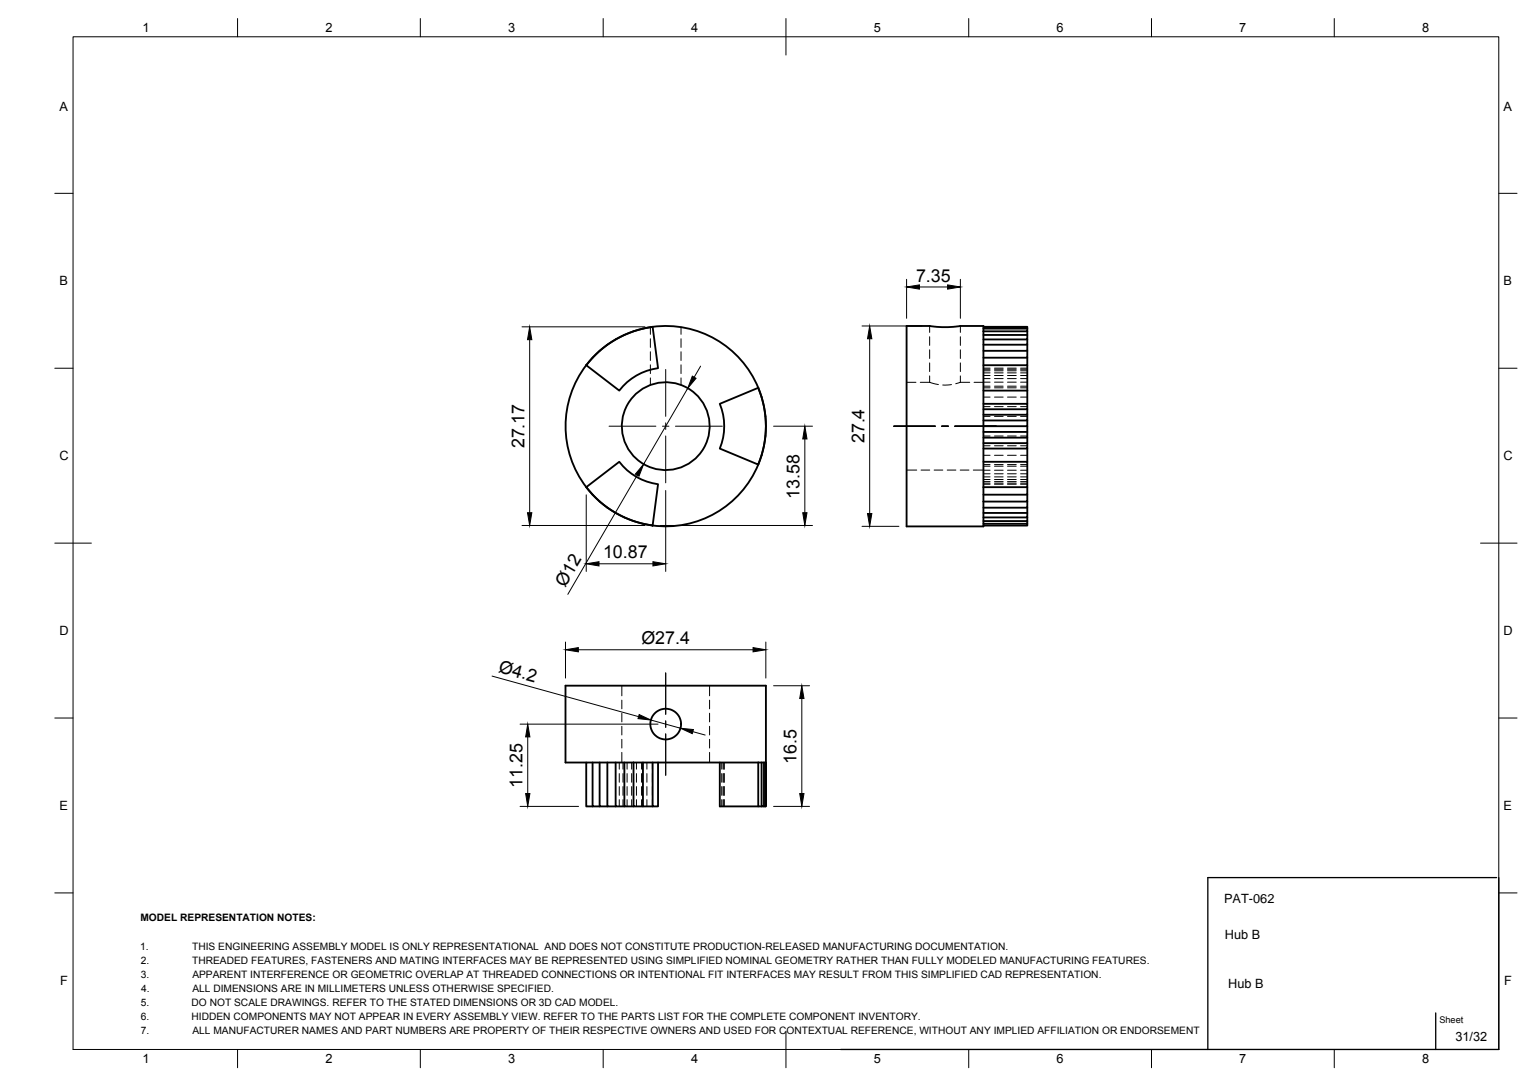
ISO-10303-21;
HEADER;
/* Generated by software containing ST-Developer
 * from STEP Tools, Inc. (www.steptools.com) 
 */

FILE_DESCRIPTION(
/* description */ ('Jaw-coupled motor to shaft test stand'),
/* implementation_level */ '2;1');

FILE_NAME(
/* name */ 'Hub B.step',
/* time_stamp */ '2026-10-27T10:46:06-07:00',
/* author */ (''),
/* organization */ (''),
/* preprocessor_version */ 'ST-DEVELOPER v20.2',
/* originating_system */ 'Autodesk Translation Framework v15.17.0.0',
/* authorisation */ '');

FILE_SCHEMA (('AUTOMOTIVE_DESIGN { 1 0 10303 214 3 1 1 }'));
ENDSEC;

DATA;
#10=MECHANICAL_DESIGN_GEOMETRIC_PRESENTATION_REPRESENTATION('',(#368),#19361);
#270=B_SPLINE_CURVE_WITH_KNOTS('',3,(#17784,#17785,#17786,#17787,#17788,
#17789,#17790,#17791,#17792,#17793,#17794,#17795,#17796,#17797,#17798,#17799,
#17800,#17801),.UNSPECIFIED.,.F.,.F.,(4,2,2,2,2,2,2,2,4),(0.,0.0798638474423531,
0.159727694884706,0.239545993340072,0.319364291795438,0.399182590250804,
0.47900088870617,0.558864736148523,0.638728583590876),.UNSPECIFIED.);
#271=B_SPLINE_CURVE_WITH_KNOTS('',3,(#17802,#17803,#17804,#17805,#17806,
#17807,#17808,#17809,#17810,#17811,#17812,#17813,#17814,#17815,#17816,#17817,
#17818,#17819),.UNSPECIFIED.,.F.,.F.,(4,2,2,2,2,2,2,2,4),(0.638728583590876,
0.718592431033229,0.798456278475583,0.878274576930949,0.958092875386314,
1.03791117384168,1.11772947229705,1.1975933197394,1.27745716718175),
 .UNSPECIFIED.);
#272=B_SPLINE_CURVE_WITH_KNOTS('',3,(#17823,#17824,#17825,#17826,#17827,
#17828,#17829,#17830,#17831,#17832,#17833,#17834,#17835,#17836,#17837,#17838,
#17839,#17840),.UNSPECIFIED.,.F.,.F.,(4,2,2,2,2,2,2,2,4),(0.,0.079239302416133,
0.158478604832266,0.237716399152057,0.316954193471848,0.39619198779164,
0.475429782111431,0.554669084527564,0.633908386943697),.UNSPECIFIED.);
#273=B_SPLINE_CURVE_WITH_KNOTS('',3,(#17841,#17842,#17843,#17844,#17845,
#17846,#17847,#17848,#17849,#17850,#17851,#17852,#17853,#17854,#17855,#17856,
#17857,#17858),.UNSPECIFIED.,.F.,.F.,(4,2,2,2,2,2,2,2,4),(0.633908386943697,
0.71314768935983,0.792386991775963,0.871624786095754,0.950862580415545,
1.03010037473534,1.10933816905513,1.18857747147126,1.26781677388739),
 .UNSPECIFIED.);
#303=SHAPE_REPRESENTATION_RELATIONSHIP('SRR','None',#19520,#335);
#335=ADVANCED_BREP_SHAPE_REPRESENTATION('',(#399),#19356);
#368=STYLED_ITEM('',(#19739),#399);
#399=MANIFOLD_SOLID_BREP('Body1',#11014);
#510=FACE_BOUND('',#2102,.T.);
#511=FACE_BOUND('',#2129,.T.);
#512=FACE_BOUND('',#2187,.T.);
#513=FACE_BOUND('',#2189,.T.);
#777=PLANE('',#11987);
#778=PLANE('',#11988);
#779=PLANE('',#11989);
#780=PLANE('',#11990);
#781=PLANE('',#11991);
#782=PLANE('',#11992);
#783=PLANE('',#11993);
#784=PLANE('',#11994);
#785=PLANE('',#11995);
#786=PLANE('',#11996);
#787=PLANE('',#11997);
#788=PLANE('',#11998);
#789=PLANE('',#11999);
#790=PLANE('',#12000);
#791=PLANE('',#12001);
#792=PLANE('',#12002);
#793=PLANE('',#12003);
#794=PLANE('',#12004);
#795=PLANE('',#12005);
#796=PLANE('',#12006);
#797=PLANE('',#12008);
#798=PLANE('',#12010);
#799=PLANE('',#12012);
#800=PLANE('',#12014);
#801=PLANE('',#12016);
#802=PLANE('',#12018);
#803=PLANE('',#12023);
#804=PLANE('',#12025);
#805=PLANE('',#12027);
#806=PLANE('',#12028);
#807=PLANE('',#12029);
#808=PLANE('',#12030);
#809=PLANE('',#12031);
#810=PLANE('',#12032);
#811=PLANE('',#12033);
#812=PLANE('',#12034);
#813=PLANE('',#12035);
#814=PLANE('',#12036);
#815=PLANE('',#12037);
#816=PLANE('',#12038);
#817=PLANE('',#12039);
#818=PLANE('',#12040);
#819=PLANE('',#12041);
#820=PLANE('',#12042);
#821=PLANE('',#12043);
#822=PLANE('',#12044);
#823=PLANE('',#12045);
#824=PLANE('',#12046);
#825=PLANE('',#12048);
#826=PLANE('',#12050);
#827=PLANE('',#12052);
#828=PLANE('',#12054);
#829=PLANE('',#12056);
#830=PLANE('',#12058);
#831=PLANE('',#12060);
#832=PLANE('',#12062);
#833=PLANE('',#12063);
#834=PLANE('',#12064);
#835=PLANE('',#12065);
#836=PLANE('',#12066);
#837=PLANE('',#12067);
#838=PLANE('',#12068);
#839=PLANE('',#12069);
#840=PLANE('',#12070);
#841=PLANE('',#12071);
#842=PLANE('',#12072);
#843=PLANE('',#12073);
#844=PLANE('',#12074);
#845=PLANE('',#12075);
#846=PLANE('',#12076);
#847=PLANE('',#12077);
#848=PLANE('',#12078);
#849=PLANE('',#12079);
#850=PLANE('',#12080);
#851=PLANE('',#12081);
#852=PLANE('',#12083);
#853=PLANE('',#12085);
#854=PLANE('',#12087);
#855=PLANE('',#12089);
#856=PLANE('',#12091);
#857=PLANE('',#12093);
#858=PLANE('',#12095);
#859=PLANE('',#12099);
#1373=FACE_OUTER_BOUND('',#2100,.T.);
#1374=FACE_OUTER_BOUND('',#2101,.T.);
#1375=FACE_OUTER_BOUND('',#2103,.T.);
#1376=FACE_OUTER_BOUND('',#2104,.T.);
#1377=FACE_OUTER_BOUND('',#2105,.T.);
#1378=FACE_OUTER_BOUND('',#2106,.T.);
#1379=FACE_OUTER_BOUND('',#2107,.T.);
#1380=FACE_OUTER_BOUND('',#2108,.T.);
#1381=FACE_OUTER_BOUND('',#2109,.T.);
#1382=FACE_OUTER_BOUND('',#2110,.T.);
#1383=FACE_OUTER_BOUND('',#2111,.T.);
#1384=FACE_OUTER_BOUND('',#2112,.T.);
#1385=FACE_OUTER_BOUND('',#2113,.T.);
#1386=FACE_OUTER_BOUND('',#2114,.T.);
#1387=FACE_OUTER_BOUND('',#2115,.T.);
#1388=FACE_OUTER_BOUND('',#2116,.T.);
#1389=FACE_OUTER_BOUND('',#2117,.T.);
#1390=FACE_OUTER_BOUND('',#2118,.T.);
#1391=FACE_OUTER_BOUND('',#2119,.T.);
#1392=FACE_OUTER_BOUND('',#2120,.T.);
#1393=FACE_OUTER_BOUND('',#2121,.T.);
#1394=FACE_OUTER_BOUND('',#2122,.T.);
#1395=FACE_OUTER_BOUND('',#2123,.T.);
#1396=FACE_OUTER_BOUND('',#2124,.T.);
#1397=FACE_OUTER_BOUND('',#2125,.T.);
#1398=FACE_OUTER_BOUND('',#2126,.T.);
#1399=FACE_OUTER_BOUND('',#2127,.T.);
#1400=FACE_OUTER_BOUND('',#2128,.T.);
#1401=FACE_OUTER_BOUND('',#2130,.T.);
#1402=FACE_OUTER_BOUND('',#2131,.T.);
#1403=FACE_OUTER_BOUND('',#2132,.T.);
#1404=FACE_OUTER_BOUND('',#2133,.T.);
#1405=FACE_OUTER_BOUND('',#2134,.T.);
#1406=FACE_OUTER_BOUND('',#2135,.T.);
#1407=FACE_OUTER_BOUND('',#2136,.T.);
#1408=FACE_OUTER_BOUND('',#2137,.T.);
#1409=FACE_OUTER_BOUND('',#2138,.T.);
#1410=FACE_OUTER_BOUND('',#2139,.T.);
#1411=FACE_OUTER_BOUND('',#2140,.T.);
#1412=FACE_OUTER_BOUND('',#2141,.T.);
#1413=FACE_OUTER_BOUND('',#2142,.T.);
#1414=FACE_OUTER_BOUND('',#2143,.T.);
#1415=FACE_OUTER_BOUND('',#2144,.T.);
#1416=FACE_OUTER_BOUND('',#2145,.T.);
#1417=FACE_OUTER_BOUND('',#2146,.T.);
#1418=FACE_OUTER_BOUND('',#2147,.T.);
#1419=FACE_OUTER_BOUND('',#2148,.T.);
#1420=FACE_OUTER_BOUND('',#2149,.T.);
#1421=FACE_OUTER_BOUND('',#2150,.T.);
#1422=FACE_OUTER_BOUND('',#2151,.T.);
#1423=FACE_OUTER_BOUND('',#2152,.T.);
#1424=FACE_OUTER_BOUND('',#2153,.T.);
#1425=FACE_OUTER_BOUND('',#2154,.T.);
#1426=FACE_OUTER_BOUND('',#2155,.T.);
#1427=FACE_OUTER_BOUND('',#2156,.T.);
#1428=FACE_OUTER_BOUND('',#2157,.T.);
#1429=FACE_OUTER_BOUND('',#2158,.T.);
#1430=FACE_OUTER_BOUND('',#2159,.T.);
#1431=FACE_OUTER_BOUND('',#2160,.T.);
#1432=FACE_OUTER_BOUND('',#2161,.T.);
#1433=FACE_OUTER_BOUND('',#2162,.T.);
#1434=FACE_OUTER_BOUND('',#2163,.T.);
#1435=FACE_OUTER_BOUND('',#2164,.T.);
#1436=FACE_OUTER_BOUND('',#2165,.T.);
#1437=FACE_OUTER_BOUND('',#2166,.T.);
#1438=FACE_OUTER_BOUND('',#2167,.T.);
#1439=FACE_OUTER_BOUND('',#2168,.T.);
#1440=FACE_OUTER_BOUND('',#2169,.T.);
#1441=FACE_OUTER_BOUND('',#2170,.T.);
#1442=FACE_OUTER_BOUND('',#2171,.T.);
#1443=FACE_OUTER_BOUND('',#2172,.T.);
#1444=FACE_OUTER_BOUND('',#2173,.T.);
#1445=FACE_OUTER_BOUND('',#2174,.T.);
#1446=FACE_OUTER_BOUND('',#2175,.T.);
#1447=FACE_OUTER_BOUND('',#2176,.T.);
#1448=FACE_OUTER_BOUND('',#2177,.T.);
#1449=FACE_OUTER_BOUND('',#2178,.T.);
#1450=FACE_OUTER_BOUND('',#2179,.T.);
#1451=FACE_OUTER_BOUND('',#2180,.T.);
#1452=FACE_OUTER_BOUND('',#2181,.T.);
#1453=FACE_OUTER_BOUND('',#2182,.T.);
#1454=FACE_OUTER_BOUND('',#2183,.T.);
#1455=FACE_OUTER_BOUND('',#2184,.T.);
#1456=FACE_OUTER_BOUND('',#2185,.T.);
#1457=FACE_OUTER_BOUND('',#2186,.T.);
#1458=FACE_OUTER_BOUND('',#2188,.T.);
#2100=EDGE_LOOP('',(#8872,#8873,#8874,#8875,#8876,#8877));
#2101=EDGE_LOOP('',(#8878,#8879,#8880,#8881));
#2102=EDGE_LOOP('',(#8882,#8883));
#2103=EDGE_LOOP('',(#8884,#8885,#8886,#8887));
#2104=EDGE_LOOP('',(#8888,#8889,#8890,#8891));
#2105=EDGE_LOOP('',(#8892,#8893,#8894,#8895));
#2106=EDGE_LOOP('',(#8896,#8897,#8898,#8899));
#2107=EDGE_LOOP('',(#8900,#8901,#8902,#8903));
#2108=EDGE_LOOP('',(#8904,#8905,#8906,#8907));
#2109=EDGE_LOOP('',(#8908,#8909,#8910,#8911));
#2110=EDGE_LOOP('',(#8912,#8913,#8914,#8915));
#2111=EDGE_LOOP('',(#8916,#8917,#8918,#8919));
#2112=EDGE_LOOP('',(#8920,#8921,#8922,#8923));
#2113=EDGE_LOOP('',(#8924,#8925,#8926,#8927));
#2114=EDGE_LOOP('',(#8928,#8929,#8930,#8931));
#2115=EDGE_LOOP('',(#8932,#8933,#8934,#8935));
#2116=EDGE_LOOP('',(#8936,#8937,#8938,#8939));
#2117=EDGE_LOOP('',(#8940,#8941,#8942,#8943));
#2118=EDGE_LOOP('',(#8944,#8945,#8946,#8947));
#2119=EDGE_LOOP('',(#8948,#8949,#8950,#8951));
#2120=EDGE_LOOP('',(#8952,#8953,#8954,#8955));
#2121=EDGE_LOOP('',(#8956,#8957,#8958,#8959,#8960,#8961,#8962,#8963,#8964,
#8965,#8966,#8967,#8968,#8969,#8970,#8971,#8972,#8973));
#2122=EDGE_LOOP('',(#8974,#8975));
#2123=EDGE_LOOP('',(#8976,#8977));
#2124=EDGE_LOOP('',(#8978,#8979));
#2125=EDGE_LOOP('',(#8980,#8981));
#2126=EDGE_LOOP('',(#8982,#8983));
#2127=EDGE_LOOP('',(#8984,#8985));
#2128=EDGE_LOOP('',(#8986,#8987,#8988,#8989,#8990,#8991,#8992,#8993,#8994,
#8995,#8996,#8997,#8998,#8999,#9000,#9001,#9002,#9003,#9004,#9005,#9006,
#9007,#9008,#9009,#9010,#9011,#9012,#9013,#9014,#9015,#9016,#9017,#9018,
#9019));
#2129=EDGE_LOOP('',(#9020));
#2130=EDGE_LOOP('',(#9021,#9022));
#2131=EDGE_LOOP('',(#9023,#9024));
#2132=EDGE_LOOP('',(#9025,#9026,#9027,#9028));
#2133=EDGE_LOOP('',(#9029,#9030,#9031,#9032));
#2134=EDGE_LOOP('',(#9033,#9034,#9035,#9036));
#2135=EDGE_LOOP('',(#9037,#9038,#9039,#9040));
#2136=EDGE_LOOP('',(#9041,#9042,#9043,#9044));
#2137=EDGE_LOOP('',(#9045,#9046,#9047,#9048));
#2138=EDGE_LOOP('',(#9049,#9050,#9051,#9052));
#2139=EDGE_LOOP('',(#9053,#9054,#9055,#9056));
#2140=EDGE_LOOP('',(#9057,#9058,#9059,#9060));
#2141=EDGE_LOOP('',(#9061,#9062,#9063,#9064));
#2142=EDGE_LOOP('',(#9065,#9066,#9067,#9068));
#2143=EDGE_LOOP('',(#9069,#9070,#9071,#9072));
#2144=EDGE_LOOP('',(#9073,#9074,#9075,#9076));
#2145=EDGE_LOOP('',(#9077,#9078,#9079,#9080));
#2146=EDGE_LOOP('',(#9081,#9082,#9083,#9084));
#2147=EDGE_LOOP('',(#9085,#9086,#9087,#9088));
#2148=EDGE_LOOP('',(#9089,#9090,#9091,#9092));
#2149=EDGE_LOOP('',(#9093,#9094,#9095,#9096));
#2150=EDGE_LOOP('',(#9097,#9098,#9099,#9100,#9101,#9102,#9103,#9104,#9105,
#9106,#9107,#9108,#9109,#9110,#9111,#9112,#9113,#9114));
#2151=EDGE_LOOP('',(#9115,#9116));
#2152=EDGE_LOOP('',(#9117,#9118));
#2153=EDGE_LOOP('',(#9119,#9120));
#2154=EDGE_LOOP('',(#9121,#9122));
#2155=EDGE_LOOP('',(#9123,#9124));
#2156=EDGE_LOOP('',(#9125,#9126));
#2157=EDGE_LOOP('',(#9127,#9128));
#2158=EDGE_LOOP('',(#9129,#9130));
#2159=EDGE_LOOP('',(#9131,#9132,#9133,#9134));
#2160=EDGE_LOOP('',(#9135,#9136,#9137,#9138));
#2161=EDGE_LOOP('',(#9139,#9140,#9141,#9142));
#2162=EDGE_LOOP('',(#9143,#9144,#9145,#9146));
#2163=EDGE_LOOP('',(#9147,#9148,#9149,#9150));
#2164=EDGE_LOOP('',(#9151,#9152,#9153,#9154));
#2165=EDGE_LOOP('',(#9155,#9156,#9157,#9158));
#2166=EDGE_LOOP('',(#9159,#9160,#9161,#9162));
#2167=EDGE_LOOP('',(#9163,#9164,#9165,#9166));
#2168=EDGE_LOOP('',(#9167,#9168,#9169,#9170));
#2169=EDGE_LOOP('',(#9171,#9172,#9173,#9174));
#2170=EDGE_LOOP('',(#9175,#9176,#9177,#9178));
#2171=EDGE_LOOP('',(#9179,#9180,#9181,#9182));
#2172=EDGE_LOOP('',(#9183,#9184,#9185,#9186));
#2173=EDGE_LOOP('',(#9187,#9188,#9189,#9190));
#2174=EDGE_LOOP('',(#9191,#9192,#9193,#9194));
#2175=EDGE_LOOP('',(#9195,#9196,#9197,#9198));
#2176=EDGE_LOOP('',(#9199,#9200,#9201,#9202));
#2177=EDGE_LOOP('',(#9203,#9204,#9205,#9206,#9207,#9208,#9209,#9210,#9211,
#9212,#9213,#9214,#9215,#9216,#9217,#9218,#9219,#9220));
#2178=EDGE_LOOP('',(#9221,#9222));
#2179=EDGE_LOOP('',(#9223,#9224));
#2180=EDGE_LOOP('',(#9225,#9226));
#2181=EDGE_LOOP('',(#9227,#9228));
#2182=EDGE_LOOP('',(#9229,#9230));
#2183=EDGE_LOOP('',(#9231,#9232));
#2184=EDGE_LOOP('',(#9233,#9234));
#2185=EDGE_LOOP('',(#9235,#9236));
#2186=EDGE_LOOP('',(#9237,#9238,#9239,#9240,#9241,#9242,#9243,#9244,#9245,
#9246,#9247,#9248,#9249,#9250,#9251,#9252,#9253,#9254,#9255,#9256,#9257,
#9258,#9259,#9260,#9261,#9262,#9263,#9264,#9265,#9266,#9267));
#2187=EDGE_LOOP('',(#9268,#9269));
#2188=EDGE_LOOP('',(#9270));
#2189=EDGE_LOOP('',(#9271));
#2896=LINE('',#17821,#4049);
#2897=LINE('',#17863,#4050);
#2898=LINE('',#17868,#4051);
#2899=LINE('',#17870,#4052);
#2900=LINE('',#17872,#4053);
#2901=LINE('',#17873,#4054);
#2902=LINE('',#17876,#4055);
#2903=LINE('',#17878,#4056);
#2904=LINE('',#17879,#4057);
#2905=LINE('',#17882,#4058);
#2906=LINE('',#17884,#4059);
#2907=LINE('',#17885,#4060);
#2908=LINE('',#17888,#4061);
#2909=LINE('',#17890,#4062);
#2910=LINE('',#17891,#4063);
#2911=LINE('',#17894,#4064);
#2912=LINE('',#17896,#4065);
#2913=LINE('',#17897,#4066);
#2914=LINE('',#17900,#4067);
#2915=LINE('',#17902,#4068);
#2916=LINE('',#17903,#4069);
#2917=LINE('',#17906,#4070);
#2918=LINE('',#17908,#4071);
#2919=LINE('',#17909,#4072);
#2920=LINE('',#17912,#4073);
#2921=LINE('',#17914,#4074);
#2922=LINE('',#17915,#4075);
#2923=LINE('',#17918,#4076);
#2924=LINE('',#17920,#4077);
#2925=LINE('',#17921,#4078);
#2926=LINE('',#17924,#4079);
#2927=LINE('',#17926,#4080);
#2928=LINE('',#17927,#4081);
#2929=LINE('',#17930,#4082);
#2930=LINE('',#17932,#4083);
#2931=LINE('',#17933,#4084);
#2932=LINE('',#17936,#4085);
#2933=LINE('',#17938,#4086);
#2934=LINE('',#17939,#4087);
#2935=LINE('',#17942,#4088);
#2936=LINE('',#17944,#4089);
#2937=LINE('',#17945,#4090);
#2938=LINE('',#17948,#4091);
#2939=LINE('',#17950,#4092);
#2940=LINE('',#17951,#4093);
#2941=LINE('',#17954,#4094);
#2942=LINE('',#17956,#4095);
#2943=LINE('',#17957,#4096);
#2944=LINE('',#17960,#4097);
#2945=LINE('',#17962,#4098);
#2946=LINE('',#17963,#4099);
#2947=LINE('',#17966,#4100);
#2948=LINE('',#17968,#4101);
#2949=LINE('',#17969,#4102);
#2950=LINE('',#17971,#4103);
#2951=LINE('',#17972,#4104);
#2952=LINE('',#17992,#4105);
#2953=LINE('',#17994,#4106);
#2954=LINE('',#17996,#4107);
#2955=LINE('',#17998,#4108);
#2956=LINE('',#18000,#4109);
#2957=LINE('',#18002,#4110);
#2958=LINE('',#18004,#4111);
#2959=LINE('',#18006,#4112);
#2960=LINE('',#18008,#4113);
#2961=LINE('',#18010,#4114);
#2962=LINE('',#18014,#4115);
#2963=LINE('',#18016,#4116);
#2964=LINE('',#18018,#4117);
#2965=LINE('',#18020,#4118);
#2966=LINE('',#18022,#4119);
#2967=LINE('',#18024,#4120);
#2968=LINE('',#18026,#4121);
#2969=LINE('',#18028,#4122);
#2970=LINE('',#18030,#4123);
#2971=LINE('',#18032,#4124);
#2972=LINE('',#18041,#4125);
#2973=LINE('',#18042,#4126);
#2974=LINE('',#18043,#4127);
#2975=LINE('',#18046,#4128);
#2976=LINE('',#18047,#4129);
#2977=LINE('',#18050,#4130);
#2978=LINE('',#18051,#4131);
#2979=LINE('',#18054,#4132);
#2980=LINE('',#18055,#4133);
#2981=LINE('',#18058,#4134);
#2982=LINE('',#18059,#4135);
#2983=LINE('',#18062,#4136);
#2984=LINE('',#18063,#4137);
#2985=LINE('',#18066,#4138);
#2986=LINE('',#18067,#4139);
#2987=LINE('',#18070,#4140);
#2988=LINE('',#18071,#4141);
#2989=LINE('',#18074,#4142);
#2990=LINE('',#18075,#4143);
#2991=LINE('',#18078,#4144);
#2992=LINE('',#18080,#4145);
#2993=LINE('',#18081,#4146);
#2994=LINE('',#18084,#4147);
#2995=LINE('',#18086,#4148);
#2996=LINE('',#18087,#4149);
#2997=LINE('',#18090,#4150);
#2998=LINE('',#18092,#4151);
#2999=LINE('',#18093,#4152);
#3000=LINE('',#18096,#4153);
#3001=LINE('',#18098,#4154);
#3002=LINE('',#18099,#4155);
#3003=LINE('',#18102,#4156);
#3004=LINE('',#18104,#4157);
#3005=LINE('',#18105,#4158);
#3006=LINE('',#18108,#4159);
#3007=LINE('',#18110,#4160);
#3008=LINE('',#18111,#4161);
#3009=LINE('',#18114,#4162);
#3010=LINE('',#18116,#4163);
#3011=LINE('',#18117,#4164);
#3012=LINE('',#18120,#4165);
#3013=LINE('',#18121,#4166);
#3014=LINE('',#18122,#4167);
#3015=LINE('',#18124,#4168);
#3016=LINE('',#18145,#4169);
#3017=LINE('',#18146,#4170);
#3018=LINE('',#18147,#4171);
#3019=LINE('',#18150,#4172);
#3020=LINE('',#18151,#4173);
#3021=LINE('',#18154,#4174);
#3022=LINE('',#18155,#4175);
#3023=LINE('',#18158,#4176);
#3024=LINE('',#18159,#4177);
#3025=LINE('',#18162,#4178);
#3026=LINE('',#18163,#4179);
#3027=LINE('',#18166,#4180);
#3028=LINE('',#18167,#4181);
#3029=LINE('',#18170,#4182);
#3030=LINE('',#18171,#4183);
#3031=LINE('',#18174,#4184);
#3032=LINE('',#18175,#4185);
#3033=LINE('',#18178,#4186);
#3034=LINE('',#18179,#4187);
#3035=LINE('',#18182,#4188);
#3036=LINE('',#18184,#4189);
#3037=LINE('',#18185,#4190);
#3038=LINE('',#18188,#4191);
#3039=LINE('',#18190,#4192);
#3040=LINE('',#18191,#4193);
#3041=LINE('',#18194,#4194);
#3042=LINE('',#18196,#4195);
#3043=LINE('',#18197,#4196);
#3044=LINE('',#18200,#4197);
#3045=LINE('',#18202,#4198);
#3046=LINE('',#18203,#4199);
#3047=LINE('',#18206,#4200);
#3048=LINE('',#18208,#4201);
#3049=LINE('',#18209,#4202);
#3050=LINE('',#18212,#4203);
#3051=LINE('',#18214,#4204);
#3052=LINE('',#18215,#4205);
#3053=LINE('',#18218,#4206);
#3054=LINE('',#18220,#4207);
#3055=LINE('',#18221,#4208);
#3056=LINE('',#18224,#4209);
#3057=LINE('',#18225,#4210);
#3058=LINE('',#18226,#4211);
#3059=LINE('',#18228,#4212);
#3060=LINE('',#18249,#4213);
#4049=VECTOR('',#14083,0.21);
#4050=VECTOR('',#14088,0.6);
#4051=VECTOR('',#14093,1.);
#4052=VECTOR('',#14094,1.);
#4053=VECTOR('',#14095,1.);
#4054=VECTOR('',#14096,1.);
#4055=VECTOR('',#14099,1.);
#4056=VECTOR('',#14100,1.);
#4057=VECTOR('',#14101,1.);
#4058=VECTOR('',#14104,1.);
#4059=VECTOR('',#14105,1.);
#4060=VECTOR('',#14106,1.);
#4061=VECTOR('',#14109,1.);
#4062=VECTOR('',#14110,1.);
#4063=VECTOR('',#14111,1.);
#4064=VECTOR('',#14114,1.);
#4065=VECTOR('',#14115,1.);
#4066=VECTOR('',#14116,1.);
#4067=VECTOR('',#14119,1.);
#4068=VECTOR('',#14120,1.);
#4069=VECTOR('',#14121,1.);
#4070=VECTOR('',#14124,1.);
#4071=VECTOR('',#14125,1.);
#4072=VECTOR('',#14126,1.);
#4073=VECTOR('',#14129,1.);
#4074=VECTOR('',#14130,1.);
#4075=VECTOR('',#14131,1.);
#4076=VECTOR('',#14134,1.);
#4077=VECTOR('',#14135,1.);
#4078=VECTOR('',#14136,1.);
#4079=VECTOR('',#14139,1.);
#4080=VECTOR('',#14140,1.);
#4081=VECTOR('',#14141,1.);
#4082=VECTOR('',#14144,1.);
#4083=VECTOR('',#14145,1.);
#4084=VECTOR('',#14146,1.);
#4085=VECTOR('',#14149,1.);
#4086=VECTOR('',#14150,1.);
#4087=VECTOR('',#14151,1.);
#4088=VECTOR('',#14154,1.);
#4089=VECTOR('',#14155,1.);
#4090=VECTOR('',#14156,1.);
#4091=VECTOR('',#14159,1.);
#4092=VECTOR('',#14160,1.);
#4093=VECTOR('',#14161,1.);
#4094=VECTOR('',#14164,1.);
#4095=VECTOR('',#14165,1.);
#4096=VECTOR('',#14166,1.);
#4097=VECTOR('',#14169,1.);
#4098=VECTOR('',#14170,1.);
#4099=VECTOR('',#14171,1.);
#4100=VECTOR('',#14174,1.);
#4101=VECTOR('',#14175,1.);
#4102=VECTOR('',#14176,1.);
#4103=VECTOR('',#14179,1.);
#4104=VECTOR('',#14180,1.);
#4105=VECTOR('',#14213,1.);
#4106=VECTOR('',#14214,1.);
#4107=VECTOR('',#14215,1.);
#4108=VECTOR('',#14216,1.);
#4109=VECTOR('',#14217,1.);
#4110=VECTOR('',#14218,1.);
#4111=VECTOR('',#14219,1.);
#4112=VECTOR('',#14220,1.);
#4113=VECTOR('',#14221,1.);
#4114=VECTOR('',#14222,1.);
#4115=VECTOR('',#14225,1.);
#4116=VECTOR('',#14226,1.);
#4117=VECTOR('',#14227,1.);
#4118=VECTOR('',#14228,1.);
#4119=VECTOR('',#14229,1.);
#4120=VECTOR('',#14230,1.);
#4121=VECTOR('',#14231,1.);
#4122=VECTOR('',#14232,1.);
#4123=VECTOR('',#14233,1.);
#4124=VECTOR('',#14234,1.);
#4125=VECTOR('',#14247,1.);
#4126=VECTOR('',#14248,1.);
#4127=VECTOR('',#14249,1.);
#4128=VECTOR('',#14252,1.);
#4129=VECTOR('',#14253,1.);
#4130=VECTOR('',#14256,1.);
#4131=VECTOR('',#14257,1.);
#4132=VECTOR('',#14260,1.);
#4133=VECTOR('',#14261,1.);
#4134=VECTOR('',#14264,1.);
#4135=VECTOR('',#14265,1.);
#4136=VECTOR('',#14268,1.);
#4137=VECTOR('',#14269,1.);
#4138=VECTOR('',#14272,1.);
#4139=VECTOR('',#14273,1.);
#4140=VECTOR('',#14276,1.);
#4141=VECTOR('',#14277,1.);
#4142=VECTOR('',#14280,1.);
#4143=VECTOR('',#14281,1.);
#4144=VECTOR('',#14284,1.);
#4145=VECTOR('',#14285,1.);
#4146=VECTOR('',#14286,1.);
#4147=VECTOR('',#14289,1.);
#4148=VECTOR('',#14290,1.);
#4149=VECTOR('',#14291,1.);
#4150=VECTOR('',#14294,1.);
#4151=VECTOR('',#14295,1.);
#4152=VECTOR('',#14296,1.);
#4153=VECTOR('',#14299,1.);
#4154=VECTOR('',#14300,1.);
#4155=VECTOR('',#14301,1.);
#4156=VECTOR('',#14304,1.);
#4157=VECTOR('',#14305,1.);
#4158=VECTOR('',#14306,1.);
#4159=VECTOR('',#14309,1.);
#4160=VECTOR('',#14310,1.);
#4161=VECTOR('',#14311,1.);
#4162=VECTOR('',#14314,1.);
#4163=VECTOR('',#14315,1.);
#4164=VECTOR('',#14316,1.);
#4165=VECTOR('',#14319,1.);
#4166=VECTOR('',#14320,1.);
#4167=VECTOR('',#14321,1.);
#4168=VECTOR('',#14324,1.);
#4169=VECTOR('',#14361,1.);
#4170=VECTOR('',#14362,1.);
#4171=VECTOR('',#14363,1.);
#4172=VECTOR('',#14366,1.);
#4173=VECTOR('',#14367,1.);
#4174=VECTOR('',#14370,1.);
#4175=VECTOR('',#14371,1.);
#4176=VECTOR('',#14374,1.);
#4177=VECTOR('',#14375,1.);
#4178=VECTOR('',#14378,1.);
#4179=VECTOR('',#14379,1.);
#4180=VECTOR('',#14382,1.);
#4181=VECTOR('',#14383,1.);
#4182=VECTOR('',#14386,1.);
#4183=VECTOR('',#14387,1.);
#4184=VECTOR('',#14390,1.);
#4185=VECTOR('',#14391,1.);
#4186=VECTOR('',#14394,1.);
#4187=VECTOR('',#14395,1.);
#4188=VECTOR('',#14398,1.);
#4189=VECTOR('',#14399,1.);
#4190=VECTOR('',#14400,1.);
#4191=VECTOR('',#14403,1.);
#4192=VECTOR('',#14404,1.);
#4193=VECTOR('',#14405,1.);
#4194=VECTOR('',#14408,1.);
#4195=VECTOR('',#14409,1.);
#4196=VECTOR('',#14410,1.);
#4197=VECTOR('',#14413,1.);
#4198=VECTOR('',#14414,1.);
#4199=VECTOR('',#14415,1.);
#4200=VECTOR('',#14418,1.);
#4201=VECTOR('',#14419,1.);
#4202=VECTOR('',#14420,1.);
#4203=VECTOR('',#14423,1.);
#4204=VECTOR('',#14424,1.);
#4205=VECTOR('',#14425,1.);
#4206=VECTOR('',#14428,1.);
#4207=VECTOR('',#14429,1.);
#4208=VECTOR('',#14430,1.);
#4209=VECTOR('',#14433,1.);
#4210=VECTOR('',#14434,1.);
#4211=VECTOR('',#14435,1.);
#4212=VECTOR('',#14438,1.);
#4213=VECTOR('',#14477,1.37);
#4880=CIRCLE('',#11985,0.6);
#4881=CIRCLE('',#11986,0.6);
#4882=CIRCLE('',#12007,1.37);
#4883=CIRCLE('',#12009,1.37);
#4884=CIRCLE('',#12011,1.37);
#4885=CIRCLE('',#12013,1.37);
#4886=CIRCLE('',#12015,1.37);
#4887=CIRCLE('',#12017,1.37);
#4888=CIRCLE('',#12019,1.37);
#4889=CIRCLE('',#12020,1.37);
#4890=CIRCLE('',#12021,1.37);
#4891=CIRCLE('',#12022,1.37);
#4892=CIRCLE('',#12024,1.37);
#4893=CIRCLE('',#12026,1.37);
#4894=CIRCLE('',#12047,1.37);
#4895=CIRCLE('',#12049,1.37);
#4896=CIRCLE('',#12051,1.37);
#4897=CIRCLE('',#12053,1.37);
#4898=CIRCLE('',#12055,1.37);
#4899=CIRCLE('',#12057,1.37);
#4900=CIRCLE('',#12059,1.37);
#4901=CIRCLE('',#12061,1.37);
#4902=CIRCLE('',#12082,1.37);
#4903=CIRCLE('',#12084,1.37);
#4904=CIRCLE('',#12086,1.37);
#4905=CIRCLE('',#12088,1.37);
#4906=CIRCLE('',#12090,1.37);
#4907=CIRCLE('',#12092,1.37);
#4908=CIRCLE('',#12094,1.37);
#4909=CIRCLE('',#12096,1.37);
#4910=CIRCLE('',#12098,1.37);
#5440=VERTEX_POINT('',#17782);
#5441=VERTEX_POINT('',#17783);
#5442=VERTEX_POINT('',#17820);
#5443=VERTEX_POINT('',#17822);
#5444=VERTEX_POINT('',#17860);
#5445=VERTEX_POINT('',#17862);
#5446=VERTEX_POINT('',#17866);
#5447=VERTEX_POINT('',#17867);
#5448=VERTEX_POINT('',#17869);
#5449=VERTEX_POINT('',#17871);
#5450=VERTEX_POINT('',#17875);
#5451=VERTEX_POINT('',#17877);
#5452=VERTEX_POINT('',#17881);
#5453=VERTEX_POINT('',#17883);
#5454=VERTEX_POINT('',#17887);
#5455=VERTEX_POINT('',#17889);
#5456=VERTEX_POINT('',#17893);
#5457=VERTEX_POINT('',#17895);
#5458=VERTEX_POINT('',#17899);
#5459=VERTEX_POINT('',#17901);
#5460=VERTEX_POINT('',#17905);
#5461=VERTEX_POINT('',#17907);
#5462=VERTEX_POINT('',#17911);
#5463=VERTEX_POINT('',#17913);
#5464=VERTEX_POINT('',#17917);
#5465=VERTEX_POINT('',#17919);
#5466=VERTEX_POINT('',#17923);
#5467=VERTEX_POINT('',#17925);
#5468=VERTEX_POINT('',#17929);
#5469=VERTEX_POINT('',#17931);
#5470=VERTEX_POINT('',#17935);
#5471=VERTEX_POINT('',#17937);
#5472=VERTEX_POINT('',#17941);
#5473=VERTEX_POINT('',#17943);
#5474=VERTEX_POINT('',#17947);
#5475=VERTEX_POINT('',#17949);
#5476=VERTEX_POINT('',#17953);
#5477=VERTEX_POINT('',#17955);
#5478=VERTEX_POINT('',#17959);
#5479=VERTEX_POINT('',#17961);
#5480=VERTEX_POINT('',#17965);
#5481=VERTEX_POINT('',#17967);
#5482=VERTEX_POINT('',#17987);
#5483=VERTEX_POINT('',#17989);
#5484=VERTEX_POINT('',#17991);
#5485=VERTEX_POINT('',#17993);
#5486=VERTEX_POINT('',#17995);
#5487=VERTEX_POINT('',#17997);
#5488=VERTEX_POINT('',#17999);
#5489=VERTEX_POINT('',#18001);
#5490=VERTEX_POINT('',#18003);
#5491=VERTEX_POINT('',#18005);
#5492=VERTEX_POINT('',#18007);
#5493=VERTEX_POINT('',#18009);
#5494=VERTEX_POINT('',#18011);
#5495=VERTEX_POINT('',#18013);
#5496=VERTEX_POINT('',#18015);
#5497=VERTEX_POINT('',#18017);
#5498=VERTEX_POINT('',#18019);
#5499=VERTEX_POINT('',#18021);
#5500=VERTEX_POINT('',#18023);
#5501=VERTEX_POINT('',#18025);
#5502=VERTEX_POINT('',#18027);
#5503=VERTEX_POINT('',#18029);
#5504=VERTEX_POINT('',#18031);
#5505=VERTEX_POINT('',#18039);
#5506=VERTEX_POINT('',#18040);
#5507=VERTEX_POINT('',#18045);
#5508=VERTEX_POINT('',#18049);
#5509=VERTEX_POINT('',#18053);
#5510=VERTEX_POINT('',#18057);
#5511=VERTEX_POINT('',#18061);
#5512=VERTEX_POINT('',#18065);
#5513=VERTEX_POINT('',#18069);
#5514=VERTEX_POINT('',#18073);
#5515=VERTEX_POINT('',#18077);
#5516=VERTEX_POINT('',#18079);
#5517=VERTEX_POINT('',#18083);
#5518=VERTEX_POINT('',#18085);
#5519=VERTEX_POINT('',#18089);
#5520=VERTEX_POINT('',#18091);
#5521=VERTEX_POINT('',#18095);
#5522=VERTEX_POINT('',#18097);
#5523=VERTEX_POINT('',#18101);
#5524=VERTEX_POINT('',#18103);
#5525=VERTEX_POINT('',#18107);
#5526=VERTEX_POINT('',#18109);
#5527=VERTEX_POINT('',#18113);
#5528=VERTEX_POINT('',#18115);
#5529=VERTEX_POINT('',#18119);
#5530=VERTEX_POINT('',#18143);
#5531=VERTEX_POINT('',#18144);
#5532=VERTEX_POINT('',#18149);
#5533=VERTEX_POINT('',#18153);
#5534=VERTEX_POINT('',#18157);
#5535=VERTEX_POINT('',#18161);
#5536=VERTEX_POINT('',#18165);
#5537=VERTEX_POINT('',#18169);
#5538=VERTEX_POINT('',#18173);
#5539=VERTEX_POINT('',#18177);
#5540=VERTEX_POINT('',#18181);
#5541=VERTEX_POINT('',#18183);
#5542=VERTEX_POINT('',#18187);
#5543=VERTEX_POINT('',#18189);
#5544=VERTEX_POINT('',#18193);
#5545=VERTEX_POINT('',#18195);
#5546=VERTEX_POINT('',#18199);
#5547=VERTEX_POINT('',#18201);
#5548=VERTEX_POINT('',#18205);
#5549=VERTEX_POINT('',#18207);
#5550=VERTEX_POINT('',#18211);
#5551=VERTEX_POINT('',#18213);
#5552=VERTEX_POINT('',#18217);
#5553=VERTEX_POINT('',#18219);
#5554=VERTEX_POINT('',#18223);
#5555=VERTEX_POINT('',#18247);
#6647=EDGE_CURVE('',#5440,#5441,#270,.T.);
#6648=EDGE_CURVE('',#5441,#5440,#271,.T.);
#6649=EDGE_CURVE('',#5441,#5442,#2896,.T.);
#6650=EDGE_CURVE('',#5443,#5442,#272,.T.);
#6651=EDGE_CURVE('',#5442,#5443,#273,.T.);
#6652=EDGE_CURVE('',#5444,#5444,#4880,.T.);
#6653=EDGE_CURVE('',#5444,#5445,#2897,.T.);
#6654=EDGE_CURVE('',#5445,#5445,#4881,.T.);
#6655=EDGE_CURVE('',#5446,#5447,#2898,.T.);
#6656=EDGE_CURVE('',#5447,#5448,#2899,.T.);
#6657=EDGE_CURVE('',#5449,#5448,#2900,.T.);
#6658=EDGE_CURVE('',#5446,#5449,#2901,.T.);
#6659=EDGE_CURVE('',#5450,#5446,#2902,.T.);
#6660=EDGE_CURVE('',#5451,#5449,#2903,.T.);
#6661=EDGE_CURVE('',#5450,#5451,#2904,.T.);
#6662=EDGE_CURVE('',#5452,#5450,#2905,.T.);
#6663=EDGE_CURVE('',#5453,#5451,#2906,.T.);
#6664=EDGE_CURVE('',#5452,#5453,#2907,.T.);
#6665=EDGE_CURVE('',#5454,#5452,#2908,.T.);
#6666=EDGE_CURVE('',#5455,#5453,#2909,.T.);
#6667=EDGE_CURVE('',#5454,#5455,#2910,.T.);
#6668=EDGE_CURVE('',#5456,#5454,#2911,.T.);
#6669=EDGE_CURVE('',#5457,#5455,#2912,.T.);
#6670=EDGE_CURVE('',#5456,#5457,#2913,.T.);
#6671=EDGE_CURVE('',#5458,#5456,#2914,.T.);
#6672=EDGE_CURVE('',#5459,#5457,#2915,.T.);
#6673=EDGE_CURVE('',#5458,#5459,#2916,.T.);
#6674=EDGE_CURVE('',#5460,#5458,#2917,.T.);
#6675=EDGE_CURVE('',#5461,#5459,#2918,.T.);
#6676=EDGE_CURVE('',#5460,#5461,#2919,.T.);
#6677=EDGE_CURVE('',#5462,#5460,#2920,.T.);
#6678=EDGE_CURVE('',#5463,#5461,#2921,.T.);
#6679=EDGE_CURVE('',#5462,#5463,#2922,.T.);
#6680=EDGE_CURVE('',#5464,#5462,#2923,.T.);
#6681=EDGE_CURVE('',#5465,#5463,#2924,.T.);
#6682=EDGE_CURVE('',#5464,#5465,#2925,.T.);
#6683=EDGE_CURVE('',#5466,#5464,#2926,.T.);
#6684=EDGE_CURVE('',#5467,#5465,#2927,.T.);
#6685=EDGE_CURVE('',#5466,#5467,#2928,.T.);
#6686=EDGE_CURVE('',#5468,#5466,#2929,.T.);
#6687=EDGE_CURVE('',#5469,#5467,#2930,.T.);
#6688=EDGE_CURVE('',#5468,#5469,#2931,.T.);
#6689=EDGE_CURVE('',#5470,#5468,#2932,.T.);
#6690=EDGE_CURVE('',#5471,#5469,#2933,.T.);
#6691=EDGE_CURVE('',#5470,#5471,#2934,.T.);
#6692=EDGE_CURVE('',#5472,#5470,#2935,.T.);
#6693=EDGE_CURVE('',#5473,#5471,#2936,.T.);
#6694=EDGE_CURVE('',#5472,#5473,#2937,.T.);
#6695=EDGE_CURVE('',#5474,#5472,#2938,.T.);
#6696=EDGE_CURVE('',#5475,#5473,#2939,.T.);
#6697=EDGE_CURVE('',#5474,#5475,#2940,.T.);
#6698=EDGE_CURVE('',#5476,#5474,#2941,.T.);
#6699=EDGE_CURVE('',#5477,#5475,#2942,.T.);
#6700=EDGE_CURVE('',#5476,#5477,#2943,.T.);
#6701=EDGE_CURVE('',#5478,#5476,#2944,.T.);
#6702=EDGE_CURVE('',#5479,#5477,#2945,.T.);
#6703=EDGE_CURVE('',#5478,#5479,#2946,.T.);
#6704=EDGE_CURVE('',#5480,#5478,#2947,.T.);
#6705=EDGE_CURVE('',#5481,#5479,#2948,.T.);
#6706=EDGE_CURVE('',#5480,#5481,#2949,.T.);
#6707=EDGE_CURVE('',#5447,#5480,#2950,.T.);
#6708=EDGE_CURVE('',#5448,#5481,#2951,.T.);
#6709=EDGE_CURVE('',#5481,#5479,#4882,.T.);
#6710=EDGE_CURVE('',#5479,#5477,#4883,.T.);
#6711=EDGE_CURVE('',#5477,#5475,#4884,.T.);
#6712=EDGE_CURVE('',#5475,#5473,#4885,.T.);
#6713=EDGE_CURVE('',#5473,#5471,#4886,.T.);
#6714=EDGE_CURVE('',#5471,#5469,#4887,.T.);
#6715=EDGE_CURVE('',#5482,#5481,#4888,.T.);
#6716=EDGE_CURVE('',#5483,#5482,#4889,.T.);
#6717=EDGE_CURVE('',#5483,#5484,#2952,.T.);
#6718=EDGE_CURVE('',#5484,#5485,#2953,.T.);
#6719=EDGE_CURVE('',#5485,#5486,#2954,.T.);
#6720=EDGE_CURVE('',#5486,#5487,#2955,.T.);
#6721=EDGE_CURVE('',#5487,#5488,#2956,.T.);
#6722=EDGE_CURVE('',#5488,#5489,#2957,.T.);
#6723=EDGE_CURVE('',#5489,#5490,#2958,.T.);
#6724=EDGE_CURVE('',#5490,#5491,#2959,.T.);
#6725=EDGE_CURVE('',#5491,#5492,#2960,.T.);
#6726=EDGE_CURVE('',#5492,#5493,#2961,.T.);
#6727=EDGE_CURVE('',#5494,#5493,#4890,.T.);
#6728=EDGE_CURVE('',#5494,#5495,#2962,.T.);
#6729=EDGE_CURVE('',#5495,#5496,#2963,.T.);
#6730=EDGE_CURVE('',#5496,#5497,#2964,.T.);
#6731=EDGE_CURVE('',#5497,#5498,#2965,.T.);
#6732=EDGE_CURVE('',#5498,#5499,#2966,.T.);
#6733=EDGE_CURVE('',#5499,#5500,#2967,.T.);
#6734=EDGE_CURVE('',#5500,#5501,#2968,.T.);
#6735=EDGE_CURVE('',#5501,#5502,#2969,.T.);
#6736=EDGE_CURVE('',#5502,#5503,#2970,.T.);
#6737=EDGE_CURVE('',#5503,#5504,#2971,.T.);
#6738=EDGE_CURVE('',#5465,#5504,#4891,.T.);
#6739=EDGE_CURVE('',#5467,#5465,#4892,.T.);
#6740=EDGE_CURVE('',#5469,#5467,#4893,.T.);
#6741=EDGE_CURVE('',#5505,#5506,#2972,.T.);
#6742=EDGE_CURVE('',#5506,#5492,#2973,.T.);
#6743=EDGE_CURVE('',#5505,#5491,#2974,.T.);
#6744=EDGE_CURVE('',#5507,#5505,#2975,.T.);
#6745=EDGE_CURVE('',#5507,#5490,#2976,.T.);
#6746=EDGE_CURVE('',#5508,#5507,#2977,.T.);
#6747=EDGE_CURVE('',#5508,#5489,#2978,.T.);
#6748=EDGE_CURVE('',#5509,#5508,#2979,.T.);
#6749=EDGE_CURVE('',#5509,#5488,#2980,.T.);
#6750=EDGE_CURVE('',#5510,#5509,#2981,.T.);
#6751=EDGE_CURVE('',#5510,#5487,#2982,.T.);
#6752=EDGE_CURVE('',#5511,#5510,#2983,.T.);
#6753=EDGE_CURVE('',#5511,#5486,#2984,.T.);
#6754=EDGE_CURVE('',#5512,#5511,#2985,.T.);
#6755=EDGE_CURVE('',#5512,#5485,#2986,.T.);
#6756=EDGE_CURVE('',#5513,#5512,#2987,.T.);
#6757=EDGE_CURVE('',#5513,#5484,#2988,.T.);
#6758=EDGE_CURVE('',#5514,#5513,#2989,.T.);
#6759=EDGE_CURVE('',#5514,#5483,#2990,.T.);
#6760=EDGE_CURVE('',#5515,#5514,#2991,.T.);
#6761=EDGE_CURVE('',#5516,#5483,#2992,.T.);
#6762=EDGE_CURVE('',#5515,#5516,#2993,.T.);
#6763=EDGE_CURVE('',#5517,#5515,#2994,.T.);
#6764=EDGE_CURVE('',#5518,#5516,#2995,.T.);
#6765=EDGE_CURVE('',#5517,#5518,#2996,.T.);
#6766=EDGE_CURVE('',#5519,#5517,#2997,.T.);
#6767=EDGE_CURVE('',#5520,#5518,#2998,.T.);
#6768=EDGE_CURVE('',#5519,#5520,#2999,.T.);
#6769=EDGE_CURVE('',#5521,#5519,#3000,.T.);
#6770=EDGE_CURVE('',#5522,#5520,#3001,.T.);
#6771=EDGE_CURVE('',#5521,#5522,#3002,.T.);
#6772=EDGE_CURVE('',#5523,#5521,#3003,.T.);
#6773=EDGE_CURVE('',#5524,#5522,#3004,.T.);
#6774=EDGE_CURVE('',#5523,#5524,#3005,.T.);
#6775=EDGE_CURVE('',#5525,#5523,#3006,.T.);
#6776=EDGE_CURVE('',#5526,#5524,#3007,.T.);
#6777=EDGE_CURVE('',#5525,#5526,#3008,.T.);
#6778=EDGE_CURVE('',#5527,#5525,#3009,.T.);
#6779=EDGE_CURVE('',#5528,#5526,#3010,.T.);
#6780=EDGE_CURVE('',#5527,#5528,#3011,.T.);
#6781=EDGE_CURVE('',#5529,#5527,#3012,.T.);
#6782=EDGE_CURVE('',#5493,#5528,#3013,.T.);
#6783=EDGE_CURVE('',#5529,#5493,#3014,.T.);
#6784=EDGE_CURVE('',#5506,#5529,#3015,.T.);
#6785=EDGE_CURVE('',#5493,#5528,#4894,.T.);
#6786=EDGE_CURVE('',#5528,#5526,#4895,.T.);
#6787=EDGE_CURVE('',#5526,#5524,#4896,.T.);
#6788=EDGE_CURVE('',#5524,#5522,#4897,.T.);
#6789=EDGE_CURVE('',#5522,#5520,#4898,.T.);
#6790=EDGE_CURVE('',#5520,#5518,#4899,.T.);
#6791=EDGE_CURVE('',#5516,#5483,#4900,.T.);
#6792=EDGE_CURVE('',#5518,#5516,#4901,.T.);
#6793=EDGE_CURVE('',#5530,#5531,#3016,.T.);
#6794=EDGE_CURVE('',#5531,#5503,#3017,.T.);
#6795=EDGE_CURVE('',#5530,#5502,#3018,.T.);
#6796=EDGE_CURVE('',#5532,#5530,#3019,.T.);
#6797=EDGE_CURVE('',#5532,#5501,#3020,.T.);
#6798=EDGE_CURVE('',#5533,#5532,#3021,.T.);
#6799=EDGE_CURVE('',#5533,#5500,#3022,.T.);
#6800=EDGE_CURVE('',#5534,#5533,#3023,.T.);
#6801=EDGE_CURVE('',#5534,#5499,#3024,.T.);
#6802=EDGE_CURVE('',#5535,#5534,#3025,.T.);
#6803=EDGE_CURVE('',#5535,#5498,#3026,.T.);
#6804=EDGE_CURVE('',#5536,#5535,#3027,.T.);
#6805=EDGE_CURVE('',#5536,#5497,#3028,.T.);
#6806=EDGE_CURVE('',#5537,#5536,#3029,.T.);
#6807=EDGE_CURVE('',#5537,#5496,#3030,.T.);
#6808=EDGE_CURVE('',#5538,#5537,#3031,.T.);
#6809=EDGE_CURVE('',#5538,#5495,#3032,.T.);
#6810=EDGE_CURVE('',#5539,#5538,#3033,.T.);
#6811=EDGE_CURVE('',#5539,#5494,#3034,.T.);
#6812=EDGE_CURVE('',#5540,#5539,#3035,.T.);
#6813=EDGE_CURVE('',#5541,#5494,#3036,.T.);
#6814=EDGE_CURVE('',#5540,#5541,#3037,.T.);
#6815=EDGE_CURVE('',#5542,#5540,#3038,.T.);
#6816=EDGE_CURVE('',#5543,#5541,#3039,.T.);
#6817=EDGE_CURVE('',#5542,#5543,#3040,.T.);
#6818=EDGE_CURVE('',#5544,#5542,#3041,.T.);
#6819=EDGE_CURVE('',#5545,#5543,#3042,.T.);
#6820=EDGE_CURVE('',#5544,#5545,#3043,.T.);
#6821=EDGE_CURVE('',#5546,#5544,#3044,.T.);
#6822=EDGE_CURVE('',#5547,#5545,#3045,.T.);
#6823=EDGE_CURVE('',#5546,#5547,#3046,.T.);
#6824=EDGE_CURVE('',#5548,#5546,#3047,.T.);
#6825=EDGE_CURVE('',#5549,#5547,#3048,.T.);
#6826=EDGE_CURVE('',#5548,#5549,#3049,.T.);
#6827=EDGE_CURVE('',#5550,#5548,#3050,.T.);
#6828=EDGE_CURVE('',#5551,#5549,#3051,.T.);
#6829=EDGE_CURVE('',#5550,#5551,#3052,.T.);
#6830=EDGE_CURVE('',#5552,#5550,#3053,.T.);
#6831=EDGE_CURVE('',#5553,#5551,#3054,.T.);
#6832=EDGE_CURVE('',#5552,#5553,#3055,.T.);
#6833=EDGE_CURVE('',#5554,#5552,#3056,.T.);
#6834=EDGE_CURVE('',#5504,#5553,#3057,.T.);
#6835=EDGE_CURVE('',#5554,#5504,#3058,.T.);
#6836=EDGE_CURVE('',#5531,#5554,#3059,.T.);
#6837=EDGE_CURVE('',#5504,#5553,#4902,.T.);
#6838=EDGE_CURVE('',#5553,#5551,#4903,.T.);
#6839=EDGE_CURVE('',#5551,#5549,#4904,.T.);
#6840=EDGE_CURVE('',#5549,#5547,#4905,.T.);
#6841=EDGE_CURVE('',#5547,#5545,#4906,.T.);
#6842=EDGE_CURVE('',#5545,#5543,#4907,.T.);
#6843=EDGE_CURVE('',#5541,#5494,#4908,.T.);
#6844=EDGE_CURVE('',#5543,#5541,#4909,.T.);
#6845=EDGE_CURVE('',#5555,#5555,#4910,.T.);
#6846=EDGE_CURVE('',#5555,#5482,#3060,.T.);
#8872=ORIENTED_EDGE('',*,*,#6647,.F.);
#8873=ORIENTED_EDGE('',*,*,#6648,.F.);
#8874=ORIENTED_EDGE('',*,*,#6649,.T.);
#8875=ORIENTED_EDGE('',*,*,#6650,.F.);
#8876=ORIENTED_EDGE('',*,*,#6651,.F.);
#8877=ORIENTED_EDGE('',*,*,#6649,.F.);
#8878=ORIENTED_EDGE('',*,*,#6652,.F.);
#8879=ORIENTED_EDGE('',*,*,#6653,.T.);
#8880=ORIENTED_EDGE('',*,*,#6654,.F.);
#8881=ORIENTED_EDGE('',*,*,#6653,.F.);
#8882=ORIENTED_EDGE('',*,*,#6647,.T.);
#8883=ORIENTED_EDGE('',*,*,#6648,.T.);
#8884=ORIENTED_EDGE('',*,*,#6655,.T.);
#8885=ORIENTED_EDGE('',*,*,#6656,.T.);
#8886=ORIENTED_EDGE('',*,*,#6657,.F.);
#8887=ORIENTED_EDGE('',*,*,#6658,.F.);
#8888=ORIENTED_EDGE('',*,*,#6659,.T.);
#8889=ORIENTED_EDGE('',*,*,#6658,.T.);
#8890=ORIENTED_EDGE('',*,*,#6660,.F.);
#8891=ORIENTED_EDGE('',*,*,#6661,.F.);
#8892=ORIENTED_EDGE('',*,*,#6662,.T.);
#8893=ORIENTED_EDGE('',*,*,#6661,.T.);
#8894=ORIENTED_EDGE('',*,*,#6663,.F.);
#8895=ORIENTED_EDGE('',*,*,#6664,.F.);
#8896=ORIENTED_EDGE('',*,*,#6665,.T.);
#8897=ORIENTED_EDGE('',*,*,#6664,.T.);
#8898=ORIENTED_EDGE('',*,*,#6666,.F.);
#8899=ORIENTED_EDGE('',*,*,#6667,.F.);
#8900=ORIENTED_EDGE('',*,*,#6668,.T.);
#8901=ORIENTED_EDGE('',*,*,#6667,.T.);
#8902=ORIENTED_EDGE('',*,*,#6669,.F.);
#8903=ORIENTED_EDGE('',*,*,#6670,.F.);
#8904=ORIENTED_EDGE('',*,*,#6671,.T.);
#8905=ORIENTED_EDGE('',*,*,#6670,.T.);
#8906=ORIENTED_EDGE('',*,*,#6672,.F.);
#8907=ORIENTED_EDGE('',*,*,#6673,.F.);
#8908=ORIENTED_EDGE('',*,*,#6674,.T.);
#8909=ORIENTED_EDGE('',*,*,#6673,.T.);
#8910=ORIENTED_EDGE('',*,*,#6675,.F.);
#8911=ORIENTED_EDGE('',*,*,#6676,.F.);
#8912=ORIENTED_EDGE('',*,*,#6677,.T.);
#8913=ORIENTED_EDGE('',*,*,#6676,.T.);
#8914=ORIENTED_EDGE('',*,*,#6678,.F.);
#8915=ORIENTED_EDGE('',*,*,#6679,.F.);
#8916=ORIENTED_EDGE('',*,*,#6680,.T.);
#8917=ORIENTED_EDGE('',*,*,#6679,.T.);
#8918=ORIENTED_EDGE('',*,*,#6681,.F.);
#8919=ORIENTED_EDGE('',*,*,#6682,.F.);
#8920=ORIENTED_EDGE('',*,*,#6683,.T.);
#8921=ORIENTED_EDGE('',*,*,#6682,.T.);
#8922=ORIENTED_EDGE('',*,*,#6684,.F.);
#8923=ORIENTED_EDGE('',*,*,#6685,.F.);
#8924=ORIENTED_EDGE('',*,*,#6686,.T.);
#8925=ORIENTED_EDGE('',*,*,#6685,.T.);
#8926=ORIENTED_EDGE('',*,*,#6687,.F.);
#8927=ORIENTED_EDGE('',*,*,#6688,.F.);
#8928=ORIENTED_EDGE('',*,*,#6689,.T.);
#8929=ORIENTED_EDGE('',*,*,#6688,.T.);
#8930=ORIENTED_EDGE('',*,*,#6690,.F.);
#8931=ORIENTED_EDGE('',*,*,#6691,.F.);
#8932=ORIENTED_EDGE('',*,*,#6692,.T.);
#8933=ORIENTED_EDGE('',*,*,#6691,.T.);
#8934=ORIENTED_EDGE('',*,*,#6693,.F.);
#8935=ORIENTED_EDGE('',*,*,#6694,.F.);
#8936=ORIENTED_EDGE('',*,*,#6695,.T.);
#8937=ORIENTED_EDGE('',*,*,#6694,.T.);
#8938=ORIENTED_EDGE('',*,*,#6696,.F.);
#8939=ORIENTED_EDGE('',*,*,#6697,.F.);
#8940=ORIENTED_EDGE('',*,*,#6698,.T.);
#8941=ORIENTED_EDGE('',*,*,#6697,.T.);
#8942=ORIENTED_EDGE('',*,*,#6699,.F.);
#8943=ORIENTED_EDGE('',*,*,#6700,.F.);
#8944=ORIENTED_EDGE('',*,*,#6701,.T.);
#8945=ORIENTED_EDGE('',*,*,#6700,.T.);
#8946=ORIENTED_EDGE('',*,*,#6702,.F.);
#8947=ORIENTED_EDGE('',*,*,#6703,.F.);
#8948=ORIENTED_EDGE('',*,*,#6704,.T.);
#8949=ORIENTED_EDGE('',*,*,#6703,.T.);
#8950=ORIENTED_EDGE('',*,*,#6705,.F.);
#8951=ORIENTED_EDGE('',*,*,#6706,.F.);
#8952=ORIENTED_EDGE('',*,*,#6707,.T.);
#8953=ORIENTED_EDGE('',*,*,#6706,.T.);
#8954=ORIENTED_EDGE('',*,*,#6708,.F.);
#8955=ORIENTED_EDGE('',*,*,#6656,.F.);
#8956=ORIENTED_EDGE('',*,*,#6707,.F.);
#8957=ORIENTED_EDGE('',*,*,#6655,.F.);
#8958=ORIENTED_EDGE('',*,*,#6659,.F.);
#8959=ORIENTED_EDGE('',*,*,#6662,.F.);
#8960=ORIENTED_EDGE('',*,*,#6665,.F.);
#8961=ORIENTED_EDGE('',*,*,#6668,.F.);
#8962=ORIENTED_EDGE('',*,*,#6671,.F.);
#8963=ORIENTED_EDGE('',*,*,#6674,.F.);
#8964=ORIENTED_EDGE('',*,*,#6677,.F.);
#8965=ORIENTED_EDGE('',*,*,#6680,.F.);
#8966=ORIENTED_EDGE('',*,*,#6683,.F.);
#8967=ORIENTED_EDGE('',*,*,#6686,.F.);
#8968=ORIENTED_EDGE('',*,*,#6689,.F.);
#8969=ORIENTED_EDGE('',*,*,#6692,.F.);
#8970=ORIENTED_EDGE('',*,*,#6695,.F.);
#8971=ORIENTED_EDGE('',*,*,#6698,.F.);
#8972=ORIENTED_EDGE('',*,*,#6701,.F.);
#8973=ORIENTED_EDGE('',*,*,#6704,.F.);
#8974=ORIENTED_EDGE('',*,*,#6705,.T.);
#8975=ORIENTED_EDGE('',*,*,#6709,.F.);
#8976=ORIENTED_EDGE('',*,*,#6702,.T.);
#8977=ORIENTED_EDGE('',*,*,#6710,.F.);
#8978=ORIENTED_EDGE('',*,*,#6699,.T.);
#8979=ORIENTED_EDGE('',*,*,#6711,.F.);
#8980=ORIENTED_EDGE('',*,*,#6696,.T.);
#8981=ORIENTED_EDGE('',*,*,#6712,.F.);
#8982=ORIENTED_EDGE('',*,*,#6693,.T.);
#8983=ORIENTED_EDGE('',*,*,#6713,.F.);
#8984=ORIENTED_EDGE('',*,*,#6690,.T.);
#8985=ORIENTED_EDGE('',*,*,#6714,.F.);
#8986=ORIENTED_EDGE('',*,*,#6681,.T.);
#8987=ORIENTED_EDGE('',*,*,#6678,.T.);
#8988=ORIENTED_EDGE('',*,*,#6675,.T.);
#8989=ORIENTED_EDGE('',*,*,#6672,.T.);
#8990=ORIENTED_EDGE('',*,*,#6669,.T.);
#8991=ORIENTED_EDGE('',*,*,#6666,.T.);
#8992=ORIENTED_EDGE('',*,*,#6663,.T.);
#8993=ORIENTED_EDGE('',*,*,#6660,.T.);
#8994=ORIENTED_EDGE('',*,*,#6657,.T.);
#8995=ORIENTED_EDGE('',*,*,#6708,.T.);
#8996=ORIENTED_EDGE('',*,*,#6715,.F.);
#8997=ORIENTED_EDGE('',*,*,#6716,.F.);
#8998=ORIENTED_EDGE('',*,*,#6717,.T.);
#8999=ORIENTED_EDGE('',*,*,#6718,.T.);
#9000=ORIENTED_EDGE('',*,*,#6719,.T.);
#9001=ORIENTED_EDGE('',*,*,#6720,.T.);
#9002=ORIENTED_EDGE('',*,*,#6721,.T.);
#9003=ORIENTED_EDGE('',*,*,#6722,.T.);
#9004=ORIENTED_EDGE('',*,*,#6723,.T.);
#9005=ORIENTED_EDGE('',*,*,#6724,.T.);
#9006=ORIENTED_EDGE('',*,*,#6725,.T.);
#9007=ORIENTED_EDGE('',*,*,#6726,.T.);
#9008=ORIENTED_EDGE('',*,*,#6727,.F.);
#9009=ORIENTED_EDGE('',*,*,#6728,.T.);
#9010=ORIENTED_EDGE('',*,*,#6729,.T.);
#9011=ORIENTED_EDGE('',*,*,#6730,.T.);
#9012=ORIENTED_EDGE('',*,*,#6731,.T.);
#9013=ORIENTED_EDGE('',*,*,#6732,.T.);
#9014=ORIENTED_EDGE('',*,*,#6733,.T.);
#9015=ORIENTED_EDGE('',*,*,#6734,.T.);
#9016=ORIENTED_EDGE('',*,*,#6735,.T.);
#9017=ORIENTED_EDGE('',*,*,#6736,.T.);
#9018=ORIENTED_EDGE('',*,*,#6737,.T.);
#9019=ORIENTED_EDGE('',*,*,#6738,.F.);
#9020=ORIENTED_EDGE('',*,*,#6652,.T.);
#9021=ORIENTED_EDGE('',*,*,#6684,.T.);
#9022=ORIENTED_EDGE('',*,*,#6739,.F.);
#9023=ORIENTED_EDGE('',*,*,#6687,.T.);
#9024=ORIENTED_EDGE('',*,*,#6740,.F.);
#9025=ORIENTED_EDGE('',*,*,#6741,.T.);
#9026=ORIENTED_EDGE('',*,*,#6742,.T.);
#9027=ORIENTED_EDGE('',*,*,#6725,.F.);
#9028=ORIENTED_EDGE('',*,*,#6743,.F.);
#9029=ORIENTED_EDGE('',*,*,#6744,.T.);
#9030=ORIENTED_EDGE('',*,*,#6743,.T.);
#9031=ORIENTED_EDGE('',*,*,#6724,.F.);
#9032=ORIENTED_EDGE('',*,*,#6745,.F.);
#9033=ORIENTED_EDGE('',*,*,#6746,.T.);
#9034=ORIENTED_EDGE('',*,*,#6745,.T.);
#9035=ORIENTED_EDGE('',*,*,#6723,.F.);
#9036=ORIENTED_EDGE('',*,*,#6747,.F.);
#9037=ORIENTED_EDGE('',*,*,#6748,.T.);
#9038=ORIENTED_EDGE('',*,*,#6747,.T.);
#9039=ORIENTED_EDGE('',*,*,#6722,.F.);
#9040=ORIENTED_EDGE('',*,*,#6749,.F.);
#9041=ORIENTED_EDGE('',*,*,#6750,.T.);
#9042=ORIENTED_EDGE('',*,*,#6749,.T.);
#9043=ORIENTED_EDGE('',*,*,#6721,.F.);
#9044=ORIENTED_EDGE('',*,*,#6751,.F.);
#9045=ORIENTED_EDGE('',*,*,#6752,.T.);
#9046=ORIENTED_EDGE('',*,*,#6751,.T.);
#9047=ORIENTED_EDGE('',*,*,#6720,.F.);
#9048=ORIENTED_EDGE('',*,*,#6753,.F.);
#9049=ORIENTED_EDGE('',*,*,#6754,.T.);
#9050=ORIENTED_EDGE('',*,*,#6753,.T.);
#9051=ORIENTED_EDGE('',*,*,#6719,.F.);
#9052=ORIENTED_EDGE('',*,*,#6755,.F.);
#9053=ORIENTED_EDGE('',*,*,#6756,.T.);
#9054=ORIENTED_EDGE('',*,*,#6755,.T.);
#9055=ORIENTED_EDGE('',*,*,#6718,.F.);
#9056=ORIENTED_EDGE('',*,*,#6757,.F.);
#9057=ORIENTED_EDGE('',*,*,#6758,.T.);
#9058=ORIENTED_EDGE('',*,*,#6757,.T.);
#9059=ORIENTED_EDGE('',*,*,#6717,.F.);
#9060=ORIENTED_EDGE('',*,*,#6759,.F.);
#9061=ORIENTED_EDGE('',*,*,#6760,.T.);
#9062=ORIENTED_EDGE('',*,*,#6759,.T.);
#9063=ORIENTED_EDGE('',*,*,#6761,.F.);
#9064=ORIENTED_EDGE('',*,*,#6762,.F.);
#9065=ORIENTED_EDGE('',*,*,#6763,.T.);
#9066=ORIENTED_EDGE('',*,*,#6762,.T.);
#9067=ORIENTED_EDGE('',*,*,#6764,.F.);
#9068=ORIENTED_EDGE('',*,*,#6765,.F.);
#9069=ORIENTED_EDGE('',*,*,#6766,.T.);
#9070=ORIENTED_EDGE('',*,*,#6765,.T.);
#9071=ORIENTED_EDGE('',*,*,#6767,.F.);
#9072=ORIENTED_EDGE('',*,*,#6768,.F.);
#9073=ORIENTED_EDGE('',*,*,#6769,.T.);
#9074=ORIENTED_EDGE('',*,*,#6768,.T.);
#9075=ORIENTED_EDGE('',*,*,#6770,.F.);
#9076=ORIENTED_EDGE('',*,*,#6771,.F.);
#9077=ORIENTED_EDGE('',*,*,#6772,.T.);
#9078=ORIENTED_EDGE('',*,*,#6771,.T.);
#9079=ORIENTED_EDGE('',*,*,#6773,.F.);
#9080=ORIENTED_EDGE('',*,*,#6774,.F.);
#9081=ORIENTED_EDGE('',*,*,#6775,.T.);
#9082=ORIENTED_EDGE('',*,*,#6774,.T.);
#9083=ORIENTED_EDGE('',*,*,#6776,.F.);
#9084=ORIENTED_EDGE('',*,*,#6777,.F.);
#9085=ORIENTED_EDGE('',*,*,#6778,.T.);
#9086=ORIENTED_EDGE('',*,*,#6777,.T.);
#9087=ORIENTED_EDGE('',*,*,#6779,.F.);
#9088=ORIENTED_EDGE('',*,*,#6780,.F.);
#9089=ORIENTED_EDGE('',*,*,#6781,.T.);
#9090=ORIENTED_EDGE('',*,*,#6780,.T.);
#9091=ORIENTED_EDGE('',*,*,#6782,.F.);
#9092=ORIENTED_EDGE('',*,*,#6783,.F.);
#9093=ORIENTED_EDGE('',*,*,#6784,.T.);
#9094=ORIENTED_EDGE('',*,*,#6783,.T.);
#9095=ORIENTED_EDGE('',*,*,#6726,.F.);
#9096=ORIENTED_EDGE('',*,*,#6742,.F.);
#9097=ORIENTED_EDGE('',*,*,#6784,.F.);
#9098=ORIENTED_EDGE('',*,*,#6741,.F.);
#9099=ORIENTED_EDGE('',*,*,#6744,.F.);
#9100=ORIENTED_EDGE('',*,*,#6746,.F.);
#9101=ORIENTED_EDGE('',*,*,#6748,.F.);
#9102=ORIENTED_EDGE('',*,*,#6750,.F.);
#9103=ORIENTED_EDGE('',*,*,#6752,.F.);
#9104=ORIENTED_EDGE('',*,*,#6754,.F.);
#9105=ORIENTED_EDGE('',*,*,#6756,.F.);
#9106=ORIENTED_EDGE('',*,*,#6758,.F.);
#9107=ORIENTED_EDGE('',*,*,#6760,.F.);
#9108=ORIENTED_EDGE('',*,*,#6763,.F.);
#9109=ORIENTED_EDGE('',*,*,#6766,.F.);
#9110=ORIENTED_EDGE('',*,*,#6769,.F.);
#9111=ORIENTED_EDGE('',*,*,#6772,.F.);
#9112=ORIENTED_EDGE('',*,*,#6775,.F.);
#9113=ORIENTED_EDGE('',*,*,#6778,.F.);
#9114=ORIENTED_EDGE('',*,*,#6781,.F.);
#9115=ORIENTED_EDGE('',*,*,#6782,.T.);
#9116=ORIENTED_EDGE('',*,*,#6785,.F.);
#9117=ORIENTED_EDGE('',*,*,#6779,.T.);
#9118=ORIENTED_EDGE('',*,*,#6786,.F.);
#9119=ORIENTED_EDGE('',*,*,#6776,.T.);
#9120=ORIENTED_EDGE('',*,*,#6787,.F.);
#9121=ORIENTED_EDGE('',*,*,#6773,.T.);
#9122=ORIENTED_EDGE('',*,*,#6788,.F.);
#9123=ORIENTED_EDGE('',*,*,#6770,.T.);
#9124=ORIENTED_EDGE('',*,*,#6789,.F.);
#9125=ORIENTED_EDGE('',*,*,#6767,.T.);
#9126=ORIENTED_EDGE('',*,*,#6790,.F.);
#9127=ORIENTED_EDGE('',*,*,#6761,.T.);
#9128=ORIENTED_EDGE('',*,*,#6791,.F.);
#9129=ORIENTED_EDGE('',*,*,#6764,.T.);
#9130=ORIENTED_EDGE('',*,*,#6792,.F.);
#9131=ORIENTED_EDGE('',*,*,#6793,.T.);
#9132=ORIENTED_EDGE('',*,*,#6794,.T.);
#9133=ORIENTED_EDGE('',*,*,#6736,.F.);
#9134=ORIENTED_EDGE('',*,*,#6795,.F.);
#9135=ORIENTED_EDGE('',*,*,#6796,.T.);
#9136=ORIENTED_EDGE('',*,*,#6795,.T.);
#9137=ORIENTED_EDGE('',*,*,#6735,.F.);
#9138=ORIENTED_EDGE('',*,*,#6797,.F.);
#9139=ORIENTED_EDGE('',*,*,#6798,.T.);
#9140=ORIENTED_EDGE('',*,*,#6797,.T.);
#9141=ORIENTED_EDGE('',*,*,#6734,.F.);
#9142=ORIENTED_EDGE('',*,*,#6799,.F.);
#9143=ORIENTED_EDGE('',*,*,#6800,.T.);
#9144=ORIENTED_EDGE('',*,*,#6799,.T.);
#9145=ORIENTED_EDGE('',*,*,#6733,.F.);
#9146=ORIENTED_EDGE('',*,*,#6801,.F.);
#9147=ORIENTED_EDGE('',*,*,#6802,.T.);
#9148=ORIENTED_EDGE('',*,*,#6801,.T.);
#9149=ORIENTED_EDGE('',*,*,#6732,.F.);
#9150=ORIENTED_EDGE('',*,*,#6803,.F.);
#9151=ORIENTED_EDGE('',*,*,#6804,.T.);
#9152=ORIENTED_EDGE('',*,*,#6803,.T.);
#9153=ORIENTED_EDGE('',*,*,#6731,.F.);
#9154=ORIENTED_EDGE('',*,*,#6805,.F.);
#9155=ORIENTED_EDGE('',*,*,#6806,.T.);
#9156=ORIENTED_EDGE('',*,*,#6805,.T.);
#9157=ORIENTED_EDGE('',*,*,#6730,.F.);
#9158=ORIENTED_EDGE('',*,*,#6807,.F.);
#9159=ORIENTED_EDGE('',*,*,#6808,.T.);
#9160=ORIENTED_EDGE('',*,*,#6807,.T.);
#9161=ORIENTED_EDGE('',*,*,#6729,.F.);
#9162=ORIENTED_EDGE('',*,*,#6809,.F.);
#9163=ORIENTED_EDGE('',*,*,#6810,.T.);
#9164=ORIENTED_EDGE('',*,*,#6809,.T.);
#9165=ORIENTED_EDGE('',*,*,#6728,.F.);
#9166=ORIENTED_EDGE('',*,*,#6811,.F.);
#9167=ORIENTED_EDGE('',*,*,#6812,.T.);
#9168=ORIENTED_EDGE('',*,*,#6811,.T.);
#9169=ORIENTED_EDGE('',*,*,#6813,.F.);
#9170=ORIENTED_EDGE('',*,*,#6814,.F.);
#9171=ORIENTED_EDGE('',*,*,#6815,.T.);
#9172=ORIENTED_EDGE('',*,*,#6814,.T.);
#9173=ORIENTED_EDGE('',*,*,#6816,.F.);
#9174=ORIENTED_EDGE('',*,*,#6817,.F.);
#9175=ORIENTED_EDGE('',*,*,#6818,.T.);
#9176=ORIENTED_EDGE('',*,*,#6817,.T.);
#9177=ORIENTED_EDGE('',*,*,#6819,.F.);
#9178=ORIENTED_EDGE('',*,*,#6820,.F.);
#9179=ORIENTED_EDGE('',*,*,#6821,.T.);
#9180=ORIENTED_EDGE('',*,*,#6820,.T.);
#9181=ORIENTED_EDGE('',*,*,#6822,.F.);
#9182=ORIENTED_EDGE('',*,*,#6823,.F.);
#9183=ORIENTED_EDGE('',*,*,#6824,.T.);
#9184=ORIENTED_EDGE('',*,*,#6823,.T.);
#9185=ORIENTED_EDGE('',*,*,#6825,.F.);
#9186=ORIENTED_EDGE('',*,*,#6826,.F.);
#9187=ORIENTED_EDGE('',*,*,#6827,.T.);
#9188=ORIENTED_EDGE('',*,*,#6826,.T.);
#9189=ORIENTED_EDGE('',*,*,#6828,.F.);
#9190=ORIENTED_EDGE('',*,*,#6829,.F.);
#9191=ORIENTED_EDGE('',*,*,#6830,.T.);
#9192=ORIENTED_EDGE('',*,*,#6829,.T.);
#9193=ORIENTED_EDGE('',*,*,#6831,.F.);
#9194=ORIENTED_EDGE('',*,*,#6832,.F.);
#9195=ORIENTED_EDGE('',*,*,#6833,.T.);
#9196=ORIENTED_EDGE('',*,*,#6832,.T.);
#9197=ORIENTED_EDGE('',*,*,#6834,.F.);
#9198=ORIENTED_EDGE('',*,*,#6835,.F.);
#9199=ORIENTED_EDGE('',*,*,#6836,.T.);
#9200=ORIENTED_EDGE('',*,*,#6835,.T.);
#9201=ORIENTED_EDGE('',*,*,#6737,.F.);
#9202=ORIENTED_EDGE('',*,*,#6794,.F.);
#9203=ORIENTED_EDGE('',*,*,#6836,.F.);
#9204=ORIENTED_EDGE('',*,*,#6793,.F.);
#9205=ORIENTED_EDGE('',*,*,#6796,.F.);
#9206=ORIENTED_EDGE('',*,*,#6798,.F.);
#9207=ORIENTED_EDGE('',*,*,#6800,.F.);
#9208=ORIENTED_EDGE('',*,*,#6802,.F.);
#9209=ORIENTED_EDGE('',*,*,#6804,.F.);
#9210=ORIENTED_EDGE('',*,*,#6806,.F.);
#9211=ORIENTED_EDGE('',*,*,#6808,.F.);
#9212=ORIENTED_EDGE('',*,*,#6810,.F.);
#9213=ORIENTED_EDGE('',*,*,#6812,.F.);
#9214=ORIENTED_EDGE('',*,*,#6815,.F.);
#9215=ORIENTED_EDGE('',*,*,#6818,.F.);
#9216=ORIENTED_EDGE('',*,*,#6821,.F.);
#9217=ORIENTED_EDGE('',*,*,#6824,.F.);
#9218=ORIENTED_EDGE('',*,*,#6827,.F.);
#9219=ORIENTED_EDGE('',*,*,#6830,.F.);
#9220=ORIENTED_EDGE('',*,*,#6833,.F.);
#9221=ORIENTED_EDGE('',*,*,#6834,.T.);
#9222=ORIENTED_EDGE('',*,*,#6837,.F.);
#9223=ORIENTED_EDGE('',*,*,#6831,.T.);
#9224=ORIENTED_EDGE('',*,*,#6838,.F.);
#9225=ORIENTED_EDGE('',*,*,#6828,.T.);
#9226=ORIENTED_EDGE('',*,*,#6839,.F.);
#9227=ORIENTED_EDGE('',*,*,#6825,.T.);
#9228=ORIENTED_EDGE('',*,*,#6840,.F.);
#9229=ORIENTED_EDGE('',*,*,#6822,.T.);
#9230=ORIENTED_EDGE('',*,*,#6841,.F.);
#9231=ORIENTED_EDGE('',*,*,#6819,.T.);
#9232=ORIENTED_EDGE('',*,*,#6842,.F.);
#9233=ORIENTED_EDGE('',*,*,#6813,.T.);
#9234=ORIENTED_EDGE('',*,*,#6843,.F.);
#9235=ORIENTED_EDGE('',*,*,#6816,.T.);
#9236=ORIENTED_EDGE('',*,*,#6844,.F.);
#9237=ORIENTED_EDGE('',*,*,#6845,.F.);
#9238=ORIENTED_EDGE('',*,*,#6846,.T.);
#9239=ORIENTED_EDGE('',*,*,#6715,.T.);
#9240=ORIENTED_EDGE('',*,*,#6709,.T.);
#9241=ORIENTED_EDGE('',*,*,#6710,.T.);
#9242=ORIENTED_EDGE('',*,*,#6711,.T.);
#9243=ORIENTED_EDGE('',*,*,#6712,.T.);
#9244=ORIENTED_EDGE('',*,*,#6713,.T.);
#9245=ORIENTED_EDGE('',*,*,#6714,.T.);
#9246=ORIENTED_EDGE('',*,*,#6740,.T.);
#9247=ORIENTED_EDGE('',*,*,#6739,.T.);
#9248=ORIENTED_EDGE('',*,*,#6738,.T.);
#9249=ORIENTED_EDGE('',*,*,#6837,.T.);
#9250=ORIENTED_EDGE('',*,*,#6838,.T.);
#9251=ORIENTED_EDGE('',*,*,#6839,.T.);
#9252=ORIENTED_EDGE('',*,*,#6840,.T.);
#9253=ORIENTED_EDGE('',*,*,#6841,.T.);
#9254=ORIENTED_EDGE('',*,*,#6842,.T.);
#9255=ORIENTED_EDGE('',*,*,#6844,.T.);
#9256=ORIENTED_EDGE('',*,*,#6843,.T.);
#9257=ORIENTED_EDGE('',*,*,#6727,.T.);
#9258=ORIENTED_EDGE('',*,*,#6785,.T.);
#9259=ORIENTED_EDGE('',*,*,#6786,.T.);
#9260=ORIENTED_EDGE('',*,*,#6787,.T.);
#9261=ORIENTED_EDGE('',*,*,#6788,.T.);
#9262=ORIENTED_EDGE('',*,*,#6789,.T.);
#9263=ORIENTED_EDGE('',*,*,#6790,.T.);
#9264=ORIENTED_EDGE('',*,*,#6792,.T.);
#9265=ORIENTED_EDGE('',*,*,#6791,.T.);
#9266=ORIENTED_EDGE('',*,*,#6716,.T.);
#9267=ORIENTED_EDGE('',*,*,#6846,.F.);
#9268=ORIENTED_EDGE('',*,*,#6650,.T.);
#9269=ORIENTED_EDGE('',*,*,#6651,.T.);
#9270=ORIENTED_EDGE('',*,*,#6845,.T.);
#9271=ORIENTED_EDGE('',*,*,#6654,.T.);
#10350=CYLINDRICAL_SURFACE('',#11983,0.21);
#10351=CYLINDRICAL_SURFACE('',#11984,0.6);
#10352=CYLINDRICAL_SURFACE('',#12097,1.37);
#10715=ADVANCED_FACE('',(#1373),#10350,.F.);
#10716=ADVANCED_FACE('',(#1374,#510),#10351,.F.);
#10717=ADVANCED_FACE('',(#1375),#777,.T.);
#10718=ADVANCED_FACE('',(#1376),#778,.T.);
#10719=ADVANCED_FACE('',(#1377),#779,.T.);
#10720=ADVANCED_FACE('',(#1378),#780,.T.);
#10721=ADVANCED_FACE('',(#1379),#781,.T.);
#10722=ADVANCED_FACE('',(#1380),#782,.T.);
#10723=ADVANCED_FACE('',(#1381),#783,.T.);
#10724=ADVANCED_FACE('',(#1382),#784,.T.);
#10725=ADVANCED_FACE('',(#1383),#785,.T.);
#10726=ADVANCED_FACE('',(#1384),#786,.T.);
#10727=ADVANCED_FACE('',(#1385),#787,.T.);
#10728=ADVANCED_FACE('',(#1386),#788,.T.);
#10729=ADVANCED_FACE('',(#1387),#789,.T.);
#10730=ADVANCED_FACE('',(#1388),#790,.T.);
#10731=ADVANCED_FACE('',(#1389),#791,.T.);
#10732=ADVANCED_FACE('',(#1390),#792,.T.);
#10733=ADVANCED_FACE('',(#1391),#793,.T.);
#10734=ADVANCED_FACE('',(#1392),#794,.T.);
#10735=ADVANCED_FACE('',(#1393),#795,.F.);
#10736=ADVANCED_FACE('',(#1394),#796,.F.);
#10737=ADVANCED_FACE('',(#1395),#797,.F.);
#10738=ADVANCED_FACE('',(#1396),#798,.F.);
#10739=ADVANCED_FACE('',(#1397),#799,.F.);
#10740=ADVANCED_FACE('',(#1398),#800,.F.);
#10741=ADVANCED_FACE('',(#1399),#801,.F.);
#10742=ADVANCED_FACE('',(#1400,#511),#802,.F.);
#10743=ADVANCED_FACE('',(#1401),#803,.F.);
#10744=ADVANCED_FACE('',(#1402),#804,.F.);
#10745=ADVANCED_FACE('',(#1403),#805,.T.);
#10746=ADVANCED_FACE('',(#1404),#806,.T.);
#10747=ADVANCED_FACE('',(#1405),#807,.T.);
#10748=ADVANCED_FACE('',(#1406),#808,.T.);
#10749=ADVANCED_FACE('',(#1407),#809,.T.);
#10750=ADVANCED_FACE('',(#1408),#810,.T.);
#10751=ADVANCED_FACE('',(#1409),#811,.T.);
#10752=ADVANCED_FACE('',(#1410),#812,.T.);
#10753=ADVANCED_FACE('',(#1411),#813,.T.);
#10754=ADVANCED_FACE('',(#1412),#814,.T.);
#10755=ADVANCED_FACE('',(#1413),#815,.T.);
#10756=ADVANCED_FACE('',(#1414),#816,.T.);
#10757=ADVANCED_FACE('',(#1415),#817,.T.);
#10758=ADVANCED_FACE('',(#1416),#818,.T.);
#10759=ADVANCED_FACE('',(#1417),#819,.T.);
#10760=ADVANCED_FACE('',(#1418),#820,.T.);
#10761=ADVANCED_FACE('',(#1419),#821,.T.);
#10762=ADVANCED_FACE('',(#1420),#822,.T.);
#10763=ADVANCED_FACE('',(#1421),#823,.F.);
#10764=ADVANCED_FACE('',(#1422),#824,.F.);
#10765=ADVANCED_FACE('',(#1423),#825,.F.);
#10766=ADVANCED_FACE('',(#1424),#826,.F.);
#10767=ADVANCED_FACE('',(#1425),#827,.F.);
#10768=ADVANCED_FACE('',(#1426),#828,.F.);
#10769=ADVANCED_FACE('',(#1427),#829,.F.);
#10770=ADVANCED_FACE('',(#1428),#830,.F.);
#10771=ADVANCED_FACE('',(#1429),#831,.F.);
#10772=ADVANCED_FACE('',(#1430),#832,.T.);
#10773=ADVANCED_FACE('',(#1431),#833,.T.);
#10774=ADVANCED_FACE('',(#1432),#834,.T.);
#10775=ADVANCED_FACE('',(#1433),#835,.T.);
#10776=ADVANCED_FACE('',(#1434),#836,.T.);
#10777=ADVANCED_FACE('',(#1435),#837,.T.);
#10778=ADVANCED_FACE('',(#1436),#838,.T.);
#10779=ADVANCED_FACE('',(#1437),#839,.T.);
#10780=ADVANCED_FACE('',(#1438),#840,.T.);
#10781=ADVANCED_FACE('',(#1439),#841,.T.);
#10782=ADVANCED_FACE('',(#1440),#842,.T.);
#10783=ADVANCED_FACE('',(#1441),#843,.T.);
#10784=ADVANCED_FACE('',(#1442),#844,.T.);
#10785=ADVANCED_FACE('',(#1443),#845,.T.);
#10786=ADVANCED_FACE('',(#1444),#846,.T.);
#10787=ADVANCED_FACE('',(#1445),#847,.T.);
#10788=ADVANCED_FACE('',(#1446),#848,.T.);
#10789=ADVANCED_FACE('',(#1447),#849,.T.);
#10790=ADVANCED_FACE('',(#1448),#850,.F.);
#10791=ADVANCED_FACE('',(#1449),#851,.F.);
#10792=ADVANCED_FACE('',(#1450),#852,.F.);
#10793=ADVANCED_FACE('',(#1451),#853,.F.);
#10794=ADVANCED_FACE('',(#1452),#854,.F.);
#10795=ADVANCED_FACE('',(#1453),#855,.F.);
#10796=ADVANCED_FACE('',(#1454),#856,.F.);
#10797=ADVANCED_FACE('',(#1455),#857,.F.);
#10798=ADVANCED_FACE('',(#1456),#858,.F.);
#10799=ADVANCED_FACE('',(#1457,#512),#10352,.T.);
#10800=ADVANCED_FACE('',(#1458,#513),#859,.T.);
#11014=CLOSED_SHELL('',(#10715,#10716,#10717,#10718,#10719,#10720,#10721,
#10722,#10723,#10724,#10725,#10726,#10727,#10728,#10729,#10730,#10731,#10732,
#10733,#10734,#10735,#10736,#10737,#10738,#10739,#10740,#10741,#10742,#10743,
#10744,#10745,#10746,#10747,#10748,#10749,#10750,#10751,#10752,#10753,#10754,
#10755,#10756,#10757,#10758,#10759,#10760,#10761,#10762,#10763,#10764,#10765,
#10766,#10767,#10768,#10769,#10770,#10771,#10772,#10773,#10774,#10775,#10776,
#10777,#10778,#10779,#10780,#10781,#10782,#10783,#10784,#10785,#10786,#10787,
#10788,#10789,#10790,#10791,#10792,#10793,#10794,#10795,#10796,#10797,#10798,
#10799,#10800));
#11982=AXIS2_PLACEMENT_3D('',#17780,#14079,#14080);
#11983=AXIS2_PLACEMENT_3D('',#17781,#14081,#14082);
#11984=AXIS2_PLACEMENT_3D('',#17859,#14084,#14085);
#11985=AXIS2_PLACEMENT_3D('',#17861,#14086,#14087);
#11986=AXIS2_PLACEMENT_3D('',#17864,#14089,#14090);
#11987=AXIS2_PLACEMENT_3D('',#17865,#14091,#14092);
#11988=AXIS2_PLACEMENT_3D('',#17874,#14097,#14098);
#11989=AXIS2_PLACEMENT_3D('',#17880,#14102,#14103);
#11990=AXIS2_PLACEMENT_3D('',#17886,#14107,#14108);
#11991=AXIS2_PLACEMENT_3D('',#17892,#14112,#14113);
#11992=AXIS2_PLACEMENT_3D('',#17898,#14117,#14118);
#11993=AXIS2_PLACEMENT_3D('',#17904,#14122,#14123);
#11994=AXIS2_PLACEMENT_3D('',#17910,#14127,#14128);
#11995=AXIS2_PLACEMENT_3D('',#17916,#14132,#14133);
#11996=AXIS2_PLACEMENT_3D('',#17922,#14137,#14138);
#11997=AXIS2_PLACEMENT_3D('',#17928,#14142,#14143);
#11998=AXIS2_PLACEMENT_3D('',#17934,#14147,#14148);
#11999=AXIS2_PLACEMENT_3D('',#17940,#14152,#14153);
#12000=AXIS2_PLACEMENT_3D('',#17946,#14157,#14158);
#12001=AXIS2_PLACEMENT_3D('',#17952,#14162,#14163);
#12002=AXIS2_PLACEMENT_3D('',#17958,#14167,#14168);
#12003=AXIS2_PLACEMENT_3D('',#17964,#14172,#14173);
#12004=AXIS2_PLACEMENT_3D('',#17970,#14177,#14178);
#12005=AXIS2_PLACEMENT_3D('',#17973,#14181,#14182);
#12006=AXIS2_PLACEMENT_3D('',#17974,#14183,#14184);
#12007=AXIS2_PLACEMENT_3D('',#17975,#14185,#14186);
#12008=AXIS2_PLACEMENT_3D('',#17976,#14187,#14188);
#12009=AXIS2_PLACEMENT_3D('',#17977,#14189,#14190);
#12010=AXIS2_PLACEMENT_3D('',#17978,#14191,#14192);
#12011=AXIS2_PLACEMENT_3D('',#17979,#14193,#14194);
#12012=AXIS2_PLACEMENT_3D('',#17980,#14195,#14196);
#12013=AXIS2_PLACEMENT_3D('',#17981,#14197,#14198);
#12014=AXIS2_PLACEMENT_3D('',#17982,#14199,#14200);
#12015=AXIS2_PLACEMENT_3D('',#17983,#14201,#14202);
#12016=AXIS2_PLACEMENT_3D('',#17984,#14203,#14204);
#12017=AXIS2_PLACEMENT_3D('',#17985,#14205,#14206);
#12018=AXIS2_PLACEMENT_3D('',#17986,#14207,#14208);
#12019=AXIS2_PLACEMENT_3D('',#17988,#14209,#14210);
#12020=AXIS2_PLACEMENT_3D('',#17990,#14211,#14212);
#12021=AXIS2_PLACEMENT_3D('',#18012,#14223,#14224);
#12022=AXIS2_PLACEMENT_3D('',#18033,#14235,#14236);
#12023=AXIS2_PLACEMENT_3D('',#18034,#14237,#14238);
#12024=AXIS2_PLACEMENT_3D('',#18035,#14239,#14240);
#12025=AXIS2_PLACEMENT_3D('',#18036,#14241,#14242);
#12026=AXIS2_PLACEMENT_3D('',#18037,#14243,#14244);
#12027=AXIS2_PLACEMENT_3D('',#18038,#14245,#14246);
#12028=AXIS2_PLACEMENT_3D('',#18044,#14250,#14251);
#12029=AXIS2_PLACEMENT_3D('',#18048,#14254,#14255);
#12030=AXIS2_PLACEMENT_3D('',#18052,#14258,#14259);
#12031=AXIS2_PLACEMENT_3D('',#18056,#14262,#14263);
#12032=AXIS2_PLACEMENT_3D('',#18060,#14266,#14267);
#12033=AXIS2_PLACEMENT_3D('',#18064,#14270,#14271);
#12034=AXIS2_PLACEMENT_3D('',#18068,#14274,#14275);
#12035=AXIS2_PLACEMENT_3D('',#18072,#14278,#14279);
#12036=AXIS2_PLACEMENT_3D('',#18076,#14282,#14283);
#12037=AXIS2_PLACEMENT_3D('',#18082,#14287,#14288);
#12038=AXIS2_PLACEMENT_3D('',#18088,#14292,#14293);
#12039=AXIS2_PLACEMENT_3D('',#18094,#14297,#14298);
#12040=AXIS2_PLACEMENT_3D('',#18100,#14302,#14303);
#12041=AXIS2_PLACEMENT_3D('',#18106,#14307,#14308);
#12042=AXIS2_PLACEMENT_3D('',#18112,#14312,#14313);
#12043=AXIS2_PLACEMENT_3D('',#18118,#14317,#14318);
#12044=AXIS2_PLACEMENT_3D('',#18123,#14322,#14323);
#12045=AXIS2_PLACEMENT_3D('',#18125,#14325,#14326);
#12046=AXIS2_PLACEMENT_3D('',#18126,#14327,#14328);
#12047=AXIS2_PLACEMENT_3D('',#18127,#14329,#14330);
#12048=AXIS2_PLACEMENT_3D('',#18128,#14331,#14332);
#12049=AXIS2_PLACEMENT_3D('',#18129,#14333,#14334);
#12050=AXIS2_PLACEMENT_3D('',#18130,#14335,#14336);
#12051=AXIS2_PLACEMENT_3D('',#18131,#14337,#14338);
#12052=AXIS2_PLACEMENT_3D('',#18132,#14339,#14340);
#12053=AXIS2_PLACEMENT_3D('',#18133,#14341,#14342);
#12054=AXIS2_PLACEMENT_3D('',#18134,#14343,#14344);
#12055=AXIS2_PLACEMENT_3D('',#18135,#14345,#14346);
#12056=AXIS2_PLACEMENT_3D('',#18136,#14347,#14348);
#12057=AXIS2_PLACEMENT_3D('',#18137,#14349,#14350);
#12058=AXIS2_PLACEMENT_3D('',#18138,#14351,#14352);
#12059=AXIS2_PLACEMENT_3D('',#18139,#14353,#14354);
#12060=AXIS2_PLACEMENT_3D('',#18140,#14355,#14356);
#12061=AXIS2_PLACEMENT_3D('',#18141,#14357,#14358);
#12062=AXIS2_PLACEMENT_3D('',#18142,#14359,#14360);
#12063=AXIS2_PLACEMENT_3D('',#18148,#14364,#14365);
#12064=AXIS2_PLACEMENT_3D('',#18152,#14368,#14369);
#12065=AXIS2_PLACEMENT_3D('',#18156,#14372,#14373);
#12066=AXIS2_PLACEMENT_3D('',#18160,#14376,#14377);
#12067=AXIS2_PLACEMENT_3D('',#18164,#14380,#14381);
#12068=AXIS2_PLACEMENT_3D('',#18168,#14384,#14385);
#12069=AXIS2_PLACEMENT_3D('',#18172,#14388,#14389);
#12070=AXIS2_PLACEMENT_3D('',#18176,#14392,#14393);
#12071=AXIS2_PLACEMENT_3D('',#18180,#14396,#14397);
#12072=AXIS2_PLACEMENT_3D('',#18186,#14401,#14402);
#12073=AXIS2_PLACEMENT_3D('',#18192,#14406,#14407);
#12074=AXIS2_PLACEMENT_3D('',#18198,#14411,#14412);
#12075=AXIS2_PLACEMENT_3D('',#18204,#14416,#14417);
#12076=AXIS2_PLACEMENT_3D('',#18210,#14421,#14422);
#12077=AXIS2_PLACEMENT_3D('',#18216,#14426,#14427);
#12078=AXIS2_PLACEMENT_3D('',#18222,#14431,#14432);
#12079=AXIS2_PLACEMENT_3D('',#18227,#14436,#14437);
#12080=AXIS2_PLACEMENT_3D('',#18229,#14439,#14440);
#12081=AXIS2_PLACEMENT_3D('',#18230,#14441,#14442);
#12082=AXIS2_PLACEMENT_3D('',#18231,#14443,#14444);
#12083=AXIS2_PLACEMENT_3D('',#18232,#14445,#14446);
#12084=AXIS2_PLACEMENT_3D('',#18233,#14447,#14448);
#12085=AXIS2_PLACEMENT_3D('',#18234,#14449,#14450);
#12086=AXIS2_PLACEMENT_3D('',#18235,#14451,#14452);
#12087=AXIS2_PLACEMENT_3D('',#18236,#14453,#14454);
#12088=AXIS2_PLACEMENT_3D('',#18237,#14455,#14456);
#12089=AXIS2_PLACEMENT_3D('',#18238,#14457,#14458);
#12090=AXIS2_PLACEMENT_3D('',#18239,#14459,#14460);
#12091=AXIS2_PLACEMENT_3D('',#18240,#14461,#14462);
#12092=AXIS2_PLACEMENT_3D('',#18241,#14463,#14464);
#12093=AXIS2_PLACEMENT_3D('',#18242,#14465,#14466);
#12094=AXIS2_PLACEMENT_3D('',#18243,#14467,#14468);
#12095=AXIS2_PLACEMENT_3D('',#18244,#14469,#14470);
#12096=AXIS2_PLACEMENT_3D('',#18245,#14471,#14472);
#12097=AXIS2_PLACEMENT_3D('',#18246,#14473,#14474);
#12098=AXIS2_PLACEMENT_3D('',#18248,#14475,#14476);
#12099=AXIS2_PLACEMENT_3D('',#18250,#14478,#14479);
#14079=DIRECTION('axis',(0.,0.,1.));
#14080=DIRECTION('refdir',(1.,0.,0.));
#14081=DIRECTION('center_axis',(0.866025403784439,0.,0.5));
#14082=DIRECTION('ref_axis',(0.5,0.,-0.866025403784439));
#14083=DIRECTION('',(0.866025403784439,0.,0.5));
#14084=DIRECTION('center_axis',(0.,1.,0.));
#14085=DIRECTION('ref_axis',(0.5,0.,-0.866025403784439));
#14086=DIRECTION('center_axis',(0.,1.,0.));
#14087=DIRECTION('ref_axis',(0.5,0.,-0.866025403784439));
#14088=DIRECTION('',(0.,1.,0.));
#14089=DIRECTION('center_axis',(0.,-1.,0.));
#14090=DIRECTION('ref_axis',(0.5,0.,-0.866025403784439));
#14091=DIRECTION('center_axis',(-0.179016861276632,0.,-0.983846005927078));
#14092=DIRECTION('ref_axis',(-0.983846005927078,0.,0.179016861276632));
#14093=DIRECTION('',(-0.983846005927078,0.,0.179016861276632));
#14094=DIRECTION('',(0.,1.,0.));
#14095=DIRECTION('',(-0.983846005927078,0.,0.179016861276632));
#14096=DIRECTION('',(0.,1.,0.));
#14097=DIRECTION('center_axis',(-0.274588618184931,0.,-0.961561797682962));
#14098=DIRECTION('ref_axis',(-0.961561797682962,0.,0.274588618184931));
#14099=DIRECTION('',(-0.961561797682962,0.,0.274588618184931));
#14100=DIRECTION('',(-0.961561797682962,0.,0.274588618184931));
#14101=DIRECTION('',(0.,1.,0.));
#14102=DIRECTION('center_axis',(-0.367515936594703,0.,-0.930017223684013));
#14103=DIRECTION('ref_axis',(-0.930017223684012,0.,0.367515936594703));
#14104=DIRECTION('',(-0.930017223684012,0.,0.367515936594703));
#14105=DIRECTION('',(-0.930017223684013,0.,0.367515936594703));
#14106=DIRECTION('',(0.,1.,0.));
#14107=DIRECTION('center_axis',(-0.45690387563042,0.,-0.889516075421857));
#14108=DIRECTION('ref_axis',(-0.889516075421857,0.,0.45690387563042));
#14109=DIRECTION('',(-0.889516075421857,0.,0.45690387563042));
#14110=DIRECTION('',(-0.889516075421857,0.,0.45690387563042));
#14111=DIRECTION('',(0.,1.,0.));
#14112=DIRECTION('center_axis',(-0.541891580574751,0.,-0.840448401094438));
#14113=DIRECTION('ref_axis',(-0.840448401094438,0.,0.541891580574751));
#14114=DIRECTION('',(-0.840448401094438,0.,0.541891580574751));
#14115=DIRECTION('',(-0.840448401094438,0.,0.541891580574751));
#14116=DIRECTION('',(0.,1.,0.));
#14117=DIRECTION('center_axis',(-0.621660573370077,0.,-0.783286749228651));
#14118=DIRECTION('ref_axis',(-0.783286749228651,0.,0.621660573370077));
#14119=DIRECTION('',(-0.783286749228651,0.,0.621660573370077));
#14120=DIRECTION('',(-0.783286749228651,0.,0.621660573370077));
#14121=DIRECTION('',(0.,1.,0.));
#14122=DIRECTION('center_axis',(-0.695442635009612,0.,-0.718581617779698));
#14123=DIRECTION('ref_axis',(-0.718581617779698,0.,0.695442635009612));
#14124=DIRECTION('',(-0.718581617779698,0.,0.695442635009612));
#14125=DIRECTION('',(-0.718581617779698,0.,0.695442635009612));
#14126=DIRECTION('',(0.,1.,0.));
#14127=DIRECTION('center_axis',(-0.762527203906388,0.,-0.646956152534857));
#14128=DIRECTION('ref_axis',(-0.646956152534857,0.,0.762527203906388));
#14129=DIRECTION('',(-0.646956152534858,0.,0.762527203906388));
#14130=DIRECTION('',(-0.646956152534857,0.,0.762527203906388));
#14131=DIRECTION('',(0.,1.,0.));
#14132=DIRECTION('center_axis',(0.608761429008721,0.,-0.793353340291235));
#14133=DIRECTION('ref_axis',(-0.793353340291235,0.,-0.608761429008721));
#14134=DIRECTION('',(-0.793353340291235,0.,-0.608761429008721));
#14135=DIRECTION('',(-0.793353340291235,0.,-0.608761429008721));
#14136=DIRECTION('',(0.,1.,0.));
#14137=DIRECTION('center_axis',(0.762527203906388,0.,0.646956152534857));
#14138=DIRECTION('ref_axis',(0.646956152534857,0.,-0.762527203906388));
#14139=DIRECTION('',(0.646956152534857,0.,-0.762527203906388));
#14140=DIRECTION('',(0.646956152534857,0.,-0.762527203906388));
#14141=DIRECTION('',(0.,1.,0.));
#14142=DIRECTION('center_axis',(0.695442635009612,0.,0.718581617779698));
#14143=DIRECTION('ref_axis',(0.718581617779698,0.,-0.695442635009612));
#14144=DIRECTION('',(0.718581617779698,0.,-0.695442635009612));
#14145=DIRECTION('',(0.718581617779698,0.,-0.695442635009612));
#14146=DIRECTION('',(0.,1.,0.));
#14147=DIRECTION('center_axis',(0.621660573370078,0.,0.78328674922865));
#14148=DIRECTION('ref_axis',(0.78328674922865,0.,-0.621660573370078));
#14149=DIRECTION('',(0.78328674922865,0.,-0.621660573370078));
#14150=DIRECTION('',(0.78328674922865,0.,-0.621660573370078));
#14151=DIRECTION('',(0.,1.,0.));
#14152=DIRECTION('center_axis',(0.54189158057475,0.,0.84044840109444));
#14153=DIRECTION('ref_axis',(0.84044840109444,0.,-0.54189158057475));
#14154=DIRECTION('',(0.84044840109444,0.,-0.54189158057475));
#14155=DIRECTION('',(0.84044840109444,0.,-0.54189158057475));
#14156=DIRECTION('',(0.,1.,0.));
#14157=DIRECTION('center_axis',(0.456903875630422,0.,0.889516075421856));
#14158=DIRECTION('ref_axis',(0.889516075421856,0.,-0.456903875630422));
#14159=DIRECTION('',(0.889516075421856,0.,-0.456903875630422));
#14160=DIRECTION('',(0.889516075421856,0.,-0.456903875630422));
#14161=DIRECTION('',(0.,1.,0.));
#14162=DIRECTION('center_axis',(0.367515936594702,0.,0.930017223684013));
#14163=DIRECTION('ref_axis',(0.930017223684013,0.,-0.367515936594702));
#14164=DIRECTION('',(0.930017223684013,0.,-0.367515936594702));
#14165=DIRECTION('',(0.930017223684013,0.,-0.367515936594702));
#14166=DIRECTION('',(0.,1.,0.));
#14167=DIRECTION('center_axis',(0.274588618184931,0.,0.961561797682962));
#14168=DIRECTION('ref_axis',(0.961561797682962,0.,-0.274588618184931));
#14169=DIRECTION('',(0.961561797682962,0.,-0.274588618184931));
#14170=DIRECTION('',(0.961561797682962,0.,-0.274588618184931));
#14171=DIRECTION('',(0.,1.,0.));
#14172=DIRECTION('center_axis',(0.179016861276631,0.,0.983846005927078));
#14173=DIRECTION('ref_axis',(0.983846005927078,0.,-0.179016861276631));
#14174=DIRECTION('',(0.983846005927078,0.,-0.179016861276631));
#14175=DIRECTION('',(0.983846005927078,0.,-0.179016861276631));
#14176=DIRECTION('',(0.,1.,0.));
#14177=DIRECTION('center_axis',(-0.99144486137381,0.,0.130526192220051));
#14178=DIRECTION('ref_axis',(0.130526192220051,0.,0.99144486137381));
#14179=DIRECTION('',(0.130526192220051,0.,0.99144486137381));
#14180=DIRECTION('',(0.130526192220051,0.,0.99144486137381));
#14181=DIRECTION('center_axis',(0.,1.,0.));
#14182=DIRECTION('ref_axis',(0.499999999999999,0.,0.866025403784439));
#14183=DIRECTION('center_axis',(0.,1.,0.));
#14184=DIRECTION('ref_axis',(0.5,0.,-0.866025403784439));
#14185=DIRECTION('center_axis',(0.,1.,0.));
#14186=DIRECTION('ref_axis',(0.5,0.,-0.866025403784438));
#14187=DIRECTION('center_axis',(0.,1.,0.));
#14188=DIRECTION('ref_axis',(0.5,0.,-0.866025403784439));
#14189=DIRECTION('center_axis',(0.,1.,0.));
#14190=DIRECTION('ref_axis',(0.5,0.,-0.866025403784438));
#14191=DIRECTION('center_axis',(0.,1.,0.));
#14192=DIRECTION('ref_axis',(0.5,0.,-0.866025403784439));
#14193=DIRECTION('center_axis',(0.,1.,0.));
#14194=DIRECTION('ref_axis',(0.5,0.,-0.866025403784438));
#14195=DIRECTION('center_axis',(0.,1.,0.));
#14196=DIRECTION('ref_axis',(0.5,0.,-0.866025403784439));
#14197=DIRECTION('center_axis',(0.,1.,0.));
#14198=DIRECTION('ref_axis',(0.5,0.,-0.866025403784438));
#14199=DIRECTION('center_axis',(0.,1.,0.));
#14200=DIRECTION('ref_axis',(0.5,0.,-0.866025403784439));
#14201=DIRECTION('center_axis',(0.,1.,0.));
#14202=DIRECTION('ref_axis',(0.5,0.,-0.866025403784438));
#14203=DIRECTION('center_axis',(0.,1.,0.));
#14204=DIRECTION('ref_axis',(0.5,0.,-0.866025403784439));
#14205=DIRECTION('center_axis',(0.,1.,0.));
#14206=DIRECTION('ref_axis',(0.5,0.,-0.866025403784438));
#14207=DIRECTION('center_axis',(0.,1.,0.));
#14208=DIRECTION('ref_axis',(0.5,0.,-0.866025403784439));
#14209=DIRECTION('center_axis',(0.,1.,0.));
#14210=DIRECTION('ref_axis',(0.5,0.,-0.866025403784438));
#14211=DIRECTION('center_axis',(0.,1.,0.));
#14212=DIRECTION('ref_axis',(0.5,0.,-0.866025403784438));
#14213=DIRECTION('',(0.923879532511287,0.,-0.38268343236509));
#14214=DIRECTION('',(-0.33688985339222,0.,-0.941544065183021));
#14215=DIRECTION('',(-0.242980179903264,0.,-0.970031253194544));
#14216=DIRECTION('',(-0.146730474455362,0.,-0.989176509964781));
#14217=DIRECTION('',(-0.0490676743274178,0.,-0.998795456205172));
#14218=DIRECTION('',(0.0490676743274185,0.,-0.998795456205172));
#14219=DIRECTION('',(0.146730474455362,0.,-0.989176509964781));
#14220=DIRECTION('',(0.242980179903265,0.,-0.970031253194544));
#14221=DIRECTION('',(0.336889853392221,0.,-0.941544065183021));
#14222=DIRECTION('',(-0.923879532511287,0.,-0.38268343236509));
#14223=DIRECTION('center_axis',(0.,1.,0.));
#14224=DIRECTION('ref_axis',(0.5,0.,-0.866025403784438));
#14225=DIRECTION('',(-0.130526192220052,0.,0.99144486137381));
#14226=DIRECTION('',(0.983846005927078,0.,0.179016861276632));
#14227=DIRECTION('',(0.961561797682962,0.,0.274588618184932));
#14228=DIRECTION('',(0.930017223684012,0.,0.367515936594704));
#14229=DIRECTION('',(0.889516075421856,0.,0.456903875630421));
#14230=DIRECTION('',(0.840448401094438,0.,0.541891580574752));
#14231=DIRECTION('',(0.78328674922865,0.,0.621660573370078));
#14232=DIRECTION('',(0.718581617779698,0.,0.695442635009612));
#14233=DIRECTION('',(0.646956152534857,0.,0.762527203906389));
#14234=DIRECTION('',(0.793353340291235,0.,-0.60876142900872));
#14235=DIRECTION('center_axis',(0.,1.,0.));
#14236=DIRECTION('ref_axis',(0.5,0.,-0.866025403784438));
#14237=DIRECTION('center_axis',(0.,1.,0.));
#14238=DIRECTION('ref_axis',(0.5,0.,-0.866025403784439));
#14239=DIRECTION('center_axis',(0.,1.,0.));
#14240=DIRECTION('ref_axis',(0.5,0.,-0.866025403784438));
#14241=DIRECTION('center_axis',(0.,1.,0.));
#14242=DIRECTION('ref_axis',(0.5,0.,-0.866025403784439));
#14243=DIRECTION('center_axis',(0.,1.,0.));
#14244=DIRECTION('ref_axis',(0.5,0.,-0.866025403784438));
#14245=DIRECTION('center_axis',(0.941544065183021,0.,0.336889853392221));
#14246=DIRECTION('ref_axis',(0.336889853392221,0.,-0.941544065183021));
#14247=DIRECTION('',(0.336889853392221,0.,-0.941544065183021));
#14248=DIRECTION('',(0.,1.,0.));
#14249=DIRECTION('',(0.,1.,0.));
#14250=DIRECTION('center_axis',(0.970031253194544,0.,0.242980179903265));
#14251=DIRECTION('ref_axis',(0.242980179903265,0.,-0.970031253194544));
#14252=DIRECTION('',(0.242980179903265,0.,-0.970031253194544));
#14253=DIRECTION('',(0.,1.,0.));
#14254=DIRECTION('center_axis',(0.989176509964781,0.,0.146730474455362));
#14255=DIRECTION('ref_axis',(0.146730474455362,0.,-0.989176509964781));
#14256=DIRECTION('',(0.146730474455362,0.,-0.989176509964781));
#14257=DIRECTION('',(0.,1.,0.));
#14258=DIRECTION('center_axis',(0.998795456205172,0.,0.0490676743274185));
#14259=DIRECTION('ref_axis',(0.0490676743274185,0.,-0.998795456205172));
#14260=DIRECTION('',(0.0490676743274185,0.,-0.998795456205172));
#14261=DIRECTION('',(0.,1.,0.));
#14262=DIRECTION('center_axis',(0.998795456205172,0.,-0.0490676743274178));
#14263=DIRECTION('ref_axis',(-0.0490676743274178,0.,-0.998795456205172));
#14264=DIRECTION('',(-0.0490676743274178,0.,-0.998795456205172));
#14265=DIRECTION('',(0.,1.,0.));
#14266=DIRECTION('center_axis',(0.989176509964781,0.,-0.146730474455361));
#14267=DIRECTION('ref_axis',(-0.146730474455361,0.,-0.989176509964781));
#14268=DIRECTION('',(-0.146730474455361,0.,-0.989176509964781));
#14269=DIRECTION('',(0.,1.,0.));
#14270=DIRECTION('center_axis',(0.970031253194544,0.,-0.242980179903264));
#14271=DIRECTION('ref_axis',(-0.242980179903264,0.,-0.970031253194544));
#14272=DIRECTION('',(-0.242980179903264,0.,-0.970031253194544));
#14273=DIRECTION('',(0.,1.,0.));
#14274=DIRECTION('center_axis',(0.941544065183021,0.,-0.33688985339222));
#14275=DIRECTION('ref_axis',(-0.33688985339222,0.,-0.941544065183021));
#14276=DIRECTION('',(-0.33688985339222,0.,-0.941544065183021));
#14277=DIRECTION('',(0.,1.,0.));
#14278=DIRECTION('center_axis',(0.38268343236509,0.,0.923879532511287));
#14279=DIRECTION('ref_axis',(0.923879532511287,0.,-0.38268343236509));
#14280=DIRECTION('',(0.923879532511287,0.,-0.38268343236509));
#14281=DIRECTION('',(0.,1.,0.));
#14282=DIRECTION('center_axis',(-0.941544065183021,0.,0.336889853392221));
#14283=DIRECTION('ref_axis',(0.336889853392221,0.,0.941544065183021));
#14284=DIRECTION('',(0.336889853392221,0.,0.941544065183021));
#14285=DIRECTION('',(0.336889853392221,0.,0.941544065183021));
#14286=DIRECTION('',(0.,1.,0.));
#14287=DIRECTION('center_axis',(-0.970031253194544,0.,0.242980179903264));
#14288=DIRECTION('ref_axis',(0.242980179903264,0.,0.970031253194544));
#14289=DIRECTION('',(0.242980179903264,0.,0.970031253194544));
#14290=DIRECTION('',(0.242980179903264,0.,0.970031253194544));
#14291=DIRECTION('',(0.,1.,0.));
#14292=DIRECTION('center_axis',(-0.989176509964781,0.,0.146730474455362));
#14293=DIRECTION('ref_axis',(0.146730474455362,0.,0.989176509964781));
#14294=DIRECTION('',(0.146730474455362,0.,0.989176509964781));
#14295=DIRECTION('',(0.146730474455362,0.,0.989176509964781));
#14296=DIRECTION('',(0.,1.,0.));
#14297=DIRECTION('center_axis',(-0.998795456205173,0.,0.0490676743274157));
#14298=DIRECTION('ref_axis',(0.0490676743274157,0.,0.998795456205173));
#14299=DIRECTION('',(0.0490676743274157,0.,0.998795456205173));
#14300=DIRECTION('',(0.0490676743274157,0.,0.998795456205173));
#14301=DIRECTION('',(0.,1.,0.));
#14302=DIRECTION('center_axis',(-0.998795456205173,0.,-0.0490676743274162));
#14303=DIRECTION('ref_axis',(-0.0490676743274162,0.,0.998795456205173));
#14304=DIRECTION('',(-0.0490676743274162,0.,0.998795456205173));
#14305=DIRECTION('',(-0.0490676743274162,0.,0.998795456205173));
#14306=DIRECTION('',(0.,1.,0.));
#14307=DIRECTION('center_axis',(-0.989176509964781,0.,-0.146730474455363));
#14308=DIRECTION('ref_axis',(-0.146730474455363,0.,0.989176509964781));
#14309=DIRECTION('',(-0.146730474455363,0.,0.989176509964781));
#14310=DIRECTION('',(-0.146730474455363,0.,0.989176509964781));
#14311=DIRECTION('',(0.,1.,0.));
#14312=DIRECTION('center_axis',(-0.970031253194544,0.,-0.242980179903265));
#14313=DIRECTION('ref_axis',(-0.242980179903265,0.,0.970031253194544));
#14314=DIRECTION('',(-0.242980179903265,0.,0.970031253194544));
#14315=DIRECTION('',(-0.242980179903265,0.,0.970031253194544));
#14316=DIRECTION('',(0.,1.,0.));
#14317=DIRECTION('center_axis',(-0.94154406518302,0.,-0.336889853392221));
#14318=DIRECTION('ref_axis',(-0.336889853392221,0.,0.94154406518302));
#14319=DIRECTION('',(-0.336889853392221,0.,0.94154406518302));
#14320=DIRECTION('',(-0.336889853392221,0.,0.94154406518302));
#14321=DIRECTION('',(0.,1.,0.));
#14322=DIRECTION('center_axis',(0.38268343236509,0.,-0.923879532511287));
#14323=DIRECTION('ref_axis',(-0.923879532511287,0.,-0.38268343236509));
#14324=DIRECTION('',(-0.923879532511287,0.,-0.38268343236509));
#14325=DIRECTION('center_axis',(0.,1.,0.));
#14326=DIRECTION('ref_axis',(-1.,0.,-3.33066907387547E-16));
#14327=DIRECTION('center_axis',(0.,1.,0.));
#14328=DIRECTION('ref_axis',(0.5,0.,-0.866025403784439));
#14329=DIRECTION('center_axis',(0.,1.,0.));
#14330=DIRECTION('ref_axis',(0.5,0.,-0.866025403784438));
#14331=DIRECTION('center_axis',(0.,1.,0.));
#14332=DIRECTION('ref_axis',(0.5,0.,-0.866025403784439));
#14333=DIRECTION('center_axis',(0.,1.,0.));
#14334=DIRECTION('ref_axis',(0.5,0.,-0.866025403784438));
#14335=DIRECTION('center_axis',(0.,1.,0.));
#14336=DIRECTION('ref_axis',(0.5,0.,-0.866025403784439));
#14337=DIRECTION('center_axis',(0.,1.,0.));
#14338=DIRECTION('ref_axis',(0.5,0.,-0.866025403784438));
#14339=DIRECTION('center_axis',(0.,1.,0.));
#14340=DIRECTION('ref_axis',(0.5,0.,-0.866025403784439));
#14341=DIRECTION('center_axis',(0.,1.,0.));
#14342=DIRECTION('ref_axis',(0.5,0.,-0.866025403784438));
#14343=DIRECTION('center_axis',(0.,1.,0.));
#14344=DIRECTION('ref_axis',(0.5,0.,-0.866025403784439));
#14345=DIRECTION('center_axis',(0.,1.,0.));
#14346=DIRECTION('ref_axis',(0.5,0.,-0.866025403784438));
#14347=DIRECTION('center_axis',(0.,1.,0.));
#14348=DIRECTION('ref_axis',(0.5,0.,-0.866025403784439));
#14349=DIRECTION('center_axis',(0.,1.,0.));
#14350=DIRECTION('ref_axis',(0.5,0.,-0.866025403784438));
#14351=DIRECTION('center_axis',(0.,1.,0.));
#14352=DIRECTION('ref_axis',(0.5,0.,-0.866025403784439));
#14353=DIRECTION('center_axis',(0.,1.,0.));
#14354=DIRECTION('ref_axis',(0.5,0.,-0.866025403784438));
#14355=DIRECTION('center_axis',(0.,1.,0.));
#14356=DIRECTION('ref_axis',(0.5,0.,-0.866025403784439));
#14357=DIRECTION('center_axis',(0.,1.,0.));
#14358=DIRECTION('ref_axis',(0.5,0.,-0.866025403784438));
#14359=DIRECTION('center_axis',(-0.762527203906389,0.,0.646956152534857));
#14360=DIRECTION('ref_axis',(0.646956152534857,0.,0.762527203906389));
#14361=DIRECTION('',(0.646956152534857,0.,0.762527203906389));
#14362=DIRECTION('',(0.,1.,0.));
#14363=DIRECTION('',(0.,1.,0.));
#14364=DIRECTION('center_axis',(-0.695442635009612,0.,0.718581617779698));
#14365=DIRECTION('ref_axis',(0.718581617779698,0.,0.695442635009612));
#14366=DIRECTION('',(0.718581617779698,0.,0.695442635009612));
#14367=DIRECTION('',(0.,1.,0.));
#14368=DIRECTION('center_axis',(-0.621660573370078,0.,0.78328674922865));
#14369=DIRECTION('ref_axis',(0.78328674922865,0.,0.621660573370078));
#14370=DIRECTION('',(0.78328674922865,0.,0.621660573370078));
#14371=DIRECTION('',(0.,1.,0.));
#14372=DIRECTION('center_axis',(-0.541891580574752,0.,0.840448401094438));
#14373=DIRECTION('ref_axis',(0.840448401094438,0.,0.541891580574752));
#14374=DIRECTION('',(0.840448401094438,0.,0.541891580574752));
#14375=DIRECTION('',(0.,1.,0.));
#14376=DIRECTION('center_axis',(-0.456903875630421,0.,0.889516075421856));
#14377=DIRECTION('ref_axis',(0.889516075421856,0.,0.456903875630421));
#14378=DIRECTION('',(0.889516075421856,0.,0.456903875630421));
#14379=DIRECTION('',(0.,1.,0.));
#14380=DIRECTION('center_axis',(-0.367515936594704,0.,0.930017223684012));
#14381=DIRECTION('ref_axis',(0.930017223684012,0.,0.367515936594704));
#14382=DIRECTION('',(0.930017223684012,0.,0.367515936594704));
#14383=DIRECTION('',(0.,1.,0.));
#14384=DIRECTION('center_axis',(-0.274588618184932,0.,0.961561797682962));
#14385=DIRECTION('ref_axis',(0.961561797682962,0.,0.274588618184932));
#14386=DIRECTION('',(0.961561797682962,0.,0.274588618184932));
#14387=DIRECTION('',(0.,1.,0.));
#14388=DIRECTION('center_axis',(-0.179016861276632,0.,0.983846005927078));
#14389=DIRECTION('ref_axis',(0.983846005927078,0.,0.179016861276632));
#14390=DIRECTION('',(0.983846005927077,0.,0.179016861276632));
#14391=DIRECTION('',(0.,1.,0.));
#14392=DIRECTION('center_axis',(-0.99144486137381,0.,-0.130526192220052));
#14393=DIRECTION('ref_axis',(-0.130526192220052,0.,0.99144486137381));
#14394=DIRECTION('',(-0.130526192220052,0.,0.99144486137381));
#14395=DIRECTION('',(0.,1.,0.));
#14396=DIRECTION('center_axis',(0.179016861276632,0.,-0.983846005927078));
#14397=DIRECTION('ref_axis',(-0.983846005927078,0.,-0.179016861276632));
#14398=DIRECTION('',(-0.983846005927078,0.,-0.179016861276632));
#14399=DIRECTION('',(-0.983846005927078,0.,-0.179016861276632));
#14400=DIRECTION('',(0.,1.,0.));
#14401=DIRECTION('center_axis',(0.274588618184932,0.,-0.961561797682962));
#14402=DIRECTION('ref_axis',(-0.961561797682962,0.,-0.274588618184932));
#14403=DIRECTION('',(-0.961561797682962,0.,-0.274588618184932));
#14404=DIRECTION('',(-0.961561797682962,0.,-0.274588618184932));
#14405=DIRECTION('',(0.,1.,0.));
#14406=DIRECTION('center_axis',(0.367515936594703,0.,-0.930017223684013));
#14407=DIRECTION('ref_axis',(-0.930017223684013,0.,-0.367515936594703));
#14408=DIRECTION('',(-0.930017223684013,0.,-0.367515936594703));
#14409=DIRECTION('',(-0.930017223684013,0.,-0.367515936594703));
#14410=DIRECTION('',(0.,1.,0.));
#14411=DIRECTION('center_axis',(0.456903875630423,0.,-0.889516075421855));
#14412=DIRECTION('ref_axis',(-0.889516075421855,0.,-0.456903875630423));
#14413=DIRECTION('',(-0.889516075421855,0.,-0.456903875630423));
#14414=DIRECTION('',(-0.889516075421855,0.,-0.456903875630423));
#14415=DIRECTION('',(0.,1.,0.));
#14416=DIRECTION('center_axis',(0.54189158057475,0.,-0.840448401094439));
#14417=DIRECTION('ref_axis',(-0.840448401094439,0.,-0.54189158057475));
#14418=DIRECTION('',(-0.840448401094439,0.,-0.54189158057475));
#14419=DIRECTION('',(-0.840448401094439,0.,-0.54189158057475));
#14420=DIRECTION('',(0.,1.,0.));
#14421=DIRECTION('center_axis',(0.621660573370078,0.,-0.78328674922865));
#14422=DIRECTION('ref_axis',(-0.78328674922865,0.,-0.621660573370078));
#14423=DIRECTION('',(-0.78328674922865,0.,-0.621660573370078));
#14424=DIRECTION('',(-0.78328674922865,0.,-0.621660573370078));
#14425=DIRECTION('',(0.,1.,0.));
#14426=DIRECTION('center_axis',(0.695442635009612,0.,-0.718581617779698));
#14427=DIRECTION('ref_axis',(-0.718581617779698,0.,-0.695442635009612));
#14428=DIRECTION('',(-0.718581617779698,0.,-0.695442635009612));
#14429=DIRECTION('',(-0.718581617779698,0.,-0.695442635009612));
#14430=DIRECTION('',(0.,1.,0.));
#14431=DIRECTION('center_axis',(0.762527203906389,0.,-0.646956152534857));
#14432=DIRECTION('ref_axis',(-0.646956152534857,0.,-0.762527203906389));
#14433=DIRECTION('',(-0.646956152534857,0.,-0.762527203906389));
#14434=DIRECTION('',(-0.646956152534857,0.,-0.762527203906389));
#14435=DIRECTION('',(0.,1.,0.));
#14436=DIRECTION('center_axis',(0.60876142900872,0.,0.793353340291235));
#14437=DIRECTION('ref_axis',(0.793353340291235,0.,-0.60876142900872));
#14438=DIRECTION('',(0.793353340291235,0.,-0.60876142900872));
#14439=DIRECTION('center_axis',(0.,1.,0.));
#14440=DIRECTION('ref_axis',(0.5,0.,-0.866025403784439));
#14441=DIRECTION('center_axis',(0.,1.,0.));
#14442=DIRECTION('ref_axis',(0.5,0.,-0.866025403784439));
#14443=DIRECTION('center_axis',(0.,1.,0.));
#14444=DIRECTION('ref_axis',(0.5,0.,-0.866025403784438));
#14445=DIRECTION('center_axis',(0.,1.,0.));
#14446=DIRECTION('ref_axis',(0.5,0.,-0.866025403784439));
#14447=DIRECTION('center_axis',(0.,1.,0.));
#14448=DIRECTION('ref_axis',(0.5,0.,-0.866025403784438));
#14449=DIRECTION('center_axis',(0.,1.,0.));
#14450=DIRECTION('ref_axis',(0.5,0.,-0.866025403784439));
#14451=DIRECTION('center_axis',(0.,1.,0.));
#14452=DIRECTION('ref_axis',(0.5,0.,-0.866025403784438));
#14453=DIRECTION('center_axis',(0.,1.,0.));
#14454=DIRECTION('ref_axis',(0.5,0.,-0.866025403784439));
#14455=DIRECTION('center_axis',(0.,1.,0.));
#14456=DIRECTION('ref_axis',(0.5,0.,-0.866025403784438));
#14457=DIRECTION('center_axis',(0.,1.,0.));
#14458=DIRECTION('ref_axis',(0.5,0.,-0.866025403784439));
#14459=DIRECTION('center_axis',(0.,1.,0.));
#14460=DIRECTION('ref_axis',(0.5,0.,-0.866025403784438));
#14461=DIRECTION('center_axis',(0.,1.,0.));
#14462=DIRECTION('ref_axis',(0.5,0.,-0.866025403784439));
#14463=DIRECTION('center_axis',(0.,1.,0.));
#14464=DIRECTION('ref_axis',(0.5,0.,-0.866025403784438));
#14465=DIRECTION('center_axis',(0.,1.,0.));
#14466=DIRECTION('ref_axis',(0.5,0.,-0.866025403784439));
#14467=DIRECTION('center_axis',(0.,1.,0.));
#14468=DIRECTION('ref_axis',(0.5,0.,-0.866025403784438));
#14469=DIRECTION('center_axis',(0.,1.,0.));
#14470=DIRECTION('ref_axis',(0.5,0.,-0.866025403784439));
#14471=DIRECTION('center_axis',(0.,1.,0.));
#14472=DIRECTION('ref_axis',(0.5,0.,-0.866025403784438));
#14473=DIRECTION('center_axis',(0.,1.,0.));
#14474=DIRECTION('ref_axis',(0.5,0.,-0.866025403784438));
#14475=DIRECTION('center_axis',(0.,1.,0.));
#14476=DIRECTION('ref_axis',(0.5,0.,-0.866025403784438));
#14477=DIRECTION('',(0.,-1.,0.));
#14478=DIRECTION('center_axis',(0.,1.,0.));
#14479=DIRECTION('ref_axis',(0.5,0.,-0.866025403784439));
#17780=CARTESIAN_POINT('',(0.,0.,0.));
#17781=CARTESIAN_POINT('Origin',(0.,1.525,0.));
#17782=CARTESIAN_POINT('',(0.591749422187638,1.525,0.0991595751331958));
#17783=CARTESIAN_POINT('',(0.381749422187638,1.525,0.46289024472266));
#17784=CARTESIAN_POINT('Ctrl Pts',(0.591749422187639,1.525,0.0991595751331958));
#17785=CARTESIAN_POINT('Ctrl Pts',(0.591749422187639,1.55162128248078,0.0991595751331958));
#17786=CARTESIAN_POINT('Ctrl Pts',(0.590876440724725,1.5798448972882,0.104852434209432));
#17787=CARTESIAN_POINT('Ctrl Pts',(0.586484941382362,1.63150713274392,0.127139324098885));
#17788=CARTESIAN_POINT('Ctrl Pts',(0.582861172497722,1.65496807125954,0.143660692707601));
#17789=CARTESIAN_POINT('Ctrl Pts',(0.572535383770674,1.69200621178927,0.180467056616695));
#17790=CARTESIAN_POINT('Ctrl Pts',(0.565117205136936,1.70813412776081,0.203279332063799));
#17791=CARTESIAN_POINT('Ctrl Pts',(0.545350992210601,1.72963697075952,0.251539733807139));
#17792=CARTESIAN_POINT('Ctrl Pts',(0.532918292013224,1.735,0.276958441950268));
#17793=CARTESIAN_POINT('Ctrl Pts',(0.506312192528102,1.735,0.323041558049732));
#17794=CARTESIAN_POINT('Ctrl Pts',(0.490515295643458,1.72963697075952,0.346517946329861));
#17795=CARTESIAN_POINT('Ctrl Pts',(0.45860366820005,1.70813412776081,0.387766189732349));
#17796=CARTESIAN_POINT('Ctrl Pts',(0.442556747461599,1.69200621178927,0.40559665860253));
#17797=CARTESIAN_POINT('Ctrl Pts',(0.415844395658913,1.65496807125954,0.43294223590881));
#17798=CARTESIAN_POINT('Ctrl Pts',(0.403348355180798,1.63150713274392,0.44434119612471));
#17799=CARTESIAN_POINT('Ctrl Pts',(0.386243092036367,1.5798448972882,0.459287791060626));
#17800=CARTESIAN_POINT('Ctrl Pts',(0.381749422187638,1.55162128248078,0.46289024472266));
#17801=CARTESIAN_POINT('Ctrl Pts',(0.381749422187638,1.525,0.46289024472266));
#17802=CARTESIAN_POINT('Ctrl Pts',(0.381749422187638,1.525,0.46289024472266));
#17803=CARTESIAN_POINT('Ctrl Pts',(0.381749422187638,1.49837871751922,0.46289024472266));
#17804=CARTESIAN_POINT('Ctrl Pts',(0.386243092036367,1.4701551027118,0.459287791060626));
#17805=CARTESIAN_POINT('Ctrl Pts',(0.403348355180798,1.41849286725608,0.44434119612471));
#17806=CARTESIAN_POINT('Ctrl Pts',(0.415844395658914,1.39503192874046,0.43294223590881));
#17807=CARTESIAN_POINT('Ctrl Pts',(0.442556747461599,1.35799378821073,0.40559665860253));
#17808=CARTESIAN_POINT('Ctrl Pts',(0.45860366820005,1.34186587223919,0.387766189732349));
#17809=CARTESIAN_POINT('Ctrl Pts',(0.490515295643458,1.32036302924048,0.346517946329861));
#17810=CARTESIAN_POINT('Ctrl Pts',(0.506312192528102,1.315,0.323041558049732));
#17811=CARTESIAN_POINT('Ctrl Pts',(0.532918292013224,1.315,0.276958441950268));
#17812=CARTESIAN_POINT('Ctrl Pts',(0.545350992210601,1.32036302924048,0.251539733807139));
#17813=CARTESIAN_POINT('Ctrl Pts',(0.565117205136936,1.34186587223919,0.203279332063799));
#17814=CARTESIAN_POINT('Ctrl Pts',(0.572535383770674,1.35799378821073,0.180467056616695));
#17815=CARTESIAN_POINT('Ctrl Pts',(0.582861172497722,1.39503192874046,0.143660692707601));
#17816=CARTESIAN_POINT('Ctrl Pts',(0.586484941382362,1.41849286725608,0.127139324098885));
#17817=CARTESIAN_POINT('Ctrl Pts',(0.590876440724725,1.47015510271179,0.104852434209432));
#17818=CARTESIAN_POINT('Ctrl Pts',(0.591749422187638,1.49837871751922,0.0991595751331958));
#17819=CARTESIAN_POINT('Ctrl Pts',(0.591749422187638,1.525,0.0991595751331958));
#17820=CARTESIAN_POINT('',(1.06743336697656,1.525,0.85877005482555));
#17821=CARTESIAN_POINT('',(-0.105,1.525,0.181865334794732));
#17822=CARTESIAN_POINT('',(1.27743336697656,1.525,0.495039385236086));
#17823=CARTESIAN_POINT('Ctrl Pts',(1.27743336697656,1.525,0.495039385236086));
#17824=CARTESIAN_POINT('Ctrl Pts',(1.27743336697656,1.49858689919462,0.495039385236086));
#17825=CARTESIAN_POINT('Ctrl Pts',(1.27552837579046,1.47044219200607,0.500044675653854));
#17826=CARTESIAN_POINT('Ctrl Pts',(1.26746274883014,1.41871515620915,0.520149492189153));
#17827=CARTESIAN_POINT('Ctrl Pts',(1.26126362373573,1.39512919832077,0.535224213312019));
#17828=CARTESIAN_POINT('Ctrl Pts',(1.24615878616438,1.35788630799087,0.56950781678886));
#17829=CARTESIAN_POINT('Ctrl Pts',(1.23623425750631,1.34173137598416,0.591012782176279));
#17830=CARTESIAN_POINT('Ctrl Pts',(1.213004701181,1.32028707843824,0.6373310309511));
#17831=CARTESIAN_POINT('Ctrl Pts',(1.19966110223798,1.315,0.662126019059738));
#17832=CARTESIAN_POINT('Ctrl Pts',(1.17324850413138,1.315,0.707873980940262));
#17833=CARTESIAN_POINT('Ctrl Pts',(1.15844721401428,1.32028707843824,0.731827370657151));
#17834=CARTESIAN_POINT('Ctrl Pts',(1.12994921207913,1.34173137598416,0.775103880940915));
#17835=CARTESIAN_POINT('Ctrl Pts',(1.11628763007516,1.35788630799087,0.794451257573106));
#17836=CARTESIAN_POINT('Ctrl Pts',(1.09414957731662,1.39512919832077,0.824674232368354));
#17837=CARTESIAN_POINT('Ctrl Pts',(1.08419404841645,1.41871515620915,0.837580192742778));
#17838=CARTESIAN_POINT('Ctrl Pts',(1.07081558003862,1.47044219200607,0.854617638855513));
#17839=CARTESIAN_POINT('Ctrl Pts',(1.06743336697656,1.49858689919462,0.85877005482555));
#17840=CARTESIAN_POINT('Ctrl Pts',(1.06743336697656,1.525,0.85877005482555));
#17841=CARTESIAN_POINT('Ctrl Pts',(1.06743336697656,1.525,0.85877005482555));
#17842=CARTESIAN_POINT('Ctrl Pts',(1.06743336697656,1.55141310080538,0.85877005482555));
#17843=CARTESIAN_POINT('Ctrl Pts',(1.07081558003862,1.57955780799393,0.854617638855513));
#17844=CARTESIAN_POINT('Ctrl Pts',(1.08419404841645,1.63128484379085,0.837580192742778));
#17845=CARTESIAN_POINT('Ctrl Pts',(1.09414957731662,1.65487080167923,0.824674232368354));
#17846=CARTESIAN_POINT('Ctrl Pts',(1.11628763007516,1.69211369200913,0.794451257573106));
#17847=CARTESIAN_POINT('Ctrl Pts',(1.12994921207913,1.70826862401584,0.775103880940915));
#17848=CARTESIAN_POINT('Ctrl Pts',(1.15844721401428,1.72971292156176,0.731827370657151));
#17849=CARTESIAN_POINT('Ctrl Pts',(1.17324850413138,1.735,0.707873980940262));
#17850=CARTESIAN_POINT('Ctrl Pts',(1.19966110223798,1.735,0.662126019059738));
#17851=CARTESIAN_POINT('Ctrl Pts',(1.213004701181,1.72971292156176,0.6373310309511));
#17852=CARTESIAN_POINT('Ctrl Pts',(1.23623425750631,1.70826862401584,0.591012782176279));
#17853=CARTESIAN_POINT('Ctrl Pts',(1.24615878616438,1.69211369200913,0.569507816788861));
#17854=CARTESIAN_POINT('Ctrl Pts',(1.26126362373573,1.65487080167923,0.535224213312019));
#17855=CARTESIAN_POINT('Ctrl Pts',(1.26746274883014,1.63128484379085,0.520149492189153));
#17856=CARTESIAN_POINT('Ctrl Pts',(1.27552837579046,1.57955780799392,0.500044675653854));
#17857=CARTESIAN_POINT('Ctrl Pts',(1.27743336697656,1.55141310080538,0.495039385236086));
#17858=CARTESIAN_POINT('Ctrl Pts',(1.27743336697656,1.525,0.495039385236086));
#17859=CARTESIAN_POINT('Origin',(0.,0.,0.));
#17860=CARTESIAN_POINT('',(-0.3,1.,0.519615242270663));
#17861=CARTESIAN_POINT('Origin',(0.,1.,0.));
#17862=CARTESIAN_POINT('',(-0.3,2.05,0.519615242270663));
#17863=CARTESIAN_POINT('',(-0.3,0.,0.519615242270663));
#17864=CARTESIAN_POINT('Origin',(0.,2.05,0.));
#17865=CARTESIAN_POINT('Origin',(0.181661010427498,0.4,0.779101583421867));
#17866=CARTESIAN_POINT('',(0.181661010427498,0.4,0.779101583421867));
#17867=CARTESIAN_POINT('',(0.104420953776041,0.4,0.793155889099048));
#17868=CARTESIAN_POINT('',(0.181661010427498,0.4,0.779101583421867));
#17869=CARTESIAN_POINT('',(0.104420953776041,1.,0.793155889099048));
#17870=CARTESIAN_POINT('',(0.104420953776041,0.4,0.793155889099048));
#17871=CARTESIAN_POINT('',(0.181661010427498,1.,0.779101583421867));
#17872=CARTESIAN_POINT('',(0.162350996264633,1.,0.782615159841162));
#17873=CARTESIAN_POINT('',(0.181661010427498,0.4,0.779101583421867));
#17874=CARTESIAN_POINT('Origin',(0.257151572242529,0.4,0.757544103596085));
#17875=CARTESIAN_POINT('',(0.257151572242529,0.4,0.757544103596085));
#17876=CARTESIAN_POINT('',(0.257151572242529,0.4,0.757544103596085));
#17877=CARTESIAN_POINT('',(0.257151572242529,1.,0.757544103596085));
#17878=CARTESIAN_POINT('',(0.238278931788771,1.,0.76293347355253));
#17879=CARTESIAN_POINT('',(0.257151572242529,0.4,0.757544103596085));
#17880=CARTESIAN_POINT('Origin',(0.330165623843515,0.4,0.728691059936941));
#17881=CARTESIAN_POINT('',(0.330165623843515,0.4,0.728691059936941));
#17882=CARTESIAN_POINT('',(0.330165623843515,0.4,0.728691059936941));
#17883=CARTESIAN_POINT('',(0.330165623843515,1.,0.728691059936941));
#17884=CARTESIAN_POINT('',(0.311912110943269,1.,0.735904320851727));
#17885=CARTESIAN_POINT('',(0.330165623843515,0.4,0.728691059936941));
#17886=CARTESIAN_POINT('Origin',(0.4,0.4,0.692820323027551));
#17887=CARTESIAN_POINT('',(0.4,0.4,0.692820323027551));
#17888=CARTESIAN_POINT('',(0.4,0.4,0.692820323027551));
#17889=CARTESIAN_POINT('',(0.4,1.,0.692820323027551));
#17890=CARTESIAN_POINT('',(0.382541405960878,1.,0.701788007254899));
#17891=CARTESIAN_POINT('',(0.4,0.4,0.692820323027551));
#17892=CARTESIAN_POINT('Origin',(0.465982157494241,0.4,0.650277347673292));
#17893=CARTESIAN_POINT('',(0.465982157494241,0.4,0.650277347673292));
#17894=CARTESIAN_POINT('',(0.465982157494241,0.4,0.650277347673292));
#17895=CARTESIAN_POINT('',(0.465982157494241,1.,0.650277347673292));
#17896=CARTESIAN_POINT('',(0.449486618120681,1.,0.660913091511857));
#17897=CARTESIAN_POINT('',(0.465982157494241,0.4,0.650277347673292));
#17898=CARTESIAN_POINT('Origin',(0.527476652080055,0.4,0.601471845983182));
#17899=CARTESIAN_POINT('',(0.527476652080055,0.4,0.601471845983182));
#17900=CARTESIAN_POINT('',(0.527476652080055,0.4,0.601471845983182));
#17901=CARTESIAN_POINT('',(0.527476652080055,1.,0.601471845983182));
#17902=CARTESIAN_POINT('',(0.512103028433601,1.,0.61367322140571));
#17903=CARTESIAN_POINT('',(0.527476652080055,0.4,0.601471845983182));
#17904=CARTESIAN_POINT('Origin',(0.583891258158268,0.4,0.546873841618297));
#17905=CARTESIAN_POINT('',(0.583891258158268,0.4,0.546873841618297));
#17906=CARTESIAN_POINT('',(0.583891258158268,0.4,0.546873841618297));
#17907=CARTESIAN_POINT('',(0.583891258158268,1.,0.546873841618297));
#17908=CARTESIAN_POINT('',(0.569787606638715,1.,0.560523342709519));
#17909=CARTESIAN_POINT('',(0.583891258158268,0.4,0.546873841618297));
#17910=CARTESIAN_POINT('Origin',(0.634682672232988,0.4,0.487009143206977));
#17911=CARTESIAN_POINT('',(0.634682672232988,0.4,0.487009143206977));
#17912=CARTESIAN_POINT('',(0.634682672232988,0.4,0.487009143206977));
#17913=CARTESIAN_POINT('',(0.634682672232988,1.,0.487009143206977));
#17914=CARTESIAN_POINT('',(0.621984818714308,1.,0.501975317809807));
#17915=CARTESIAN_POINT('',(0.634682672232988,0.4,0.487009143206977));
#17916=CARTESIAN_POINT('Origin',(1.08689407619899,0.4,0.834003157741948));
#17917=CARTESIAN_POINT('',(1.08689407619899,0.4,0.834003157741948));
#17918=CARTESIAN_POINT('',(1.08689407619899,0.4,0.834003157741948));
#17919=CARTESIAN_POINT('',(1.08689407619899,1.,0.834003157741948));
#17920=CARTESIAN_POINT('',(0.543447038099496,1.,0.417001578870974));
#17921=CARTESIAN_POINT('',(1.08689407619899,0.4,0.834003157741948));
#17922=CARTESIAN_POINT('Origin',(0.999913779596034,0.4,0.936521453771334));
#17923=CARTESIAN_POINT('',(0.999913779596034,0.4,0.936521453771334));
#17924=CARTESIAN_POINT('',(0.999913779596034,0.4,0.936521453771334));
#17925=CARTESIAN_POINT('',(0.999913779596034,1.,0.936521453771334));
#17926=CARTESIAN_POINT('',(1.02165885374677,1.,0.910891879763987));
#17927=CARTESIAN_POINT('',(0.999913779596034,0.4,0.936521453771334));
#17928=CARTESIAN_POINT('Origin',(0.903303766687094,0.4,1.0300205362462));
#17929=CARTESIAN_POINT('',(0.903303766687094,0.4,1.0300205362462));
#17930=CARTESIAN_POINT('',(0.903303766687094,0.4,1.0300205362462));
#17931=CARTESIAN_POINT('',(0.903303766687094,1.,1.0300205362462));
#17932=CARTESIAN_POINT('',(0.927456269914329,1.,1.00664576562748));
#17933=CARTESIAN_POINT('',(0.903303766687094,0.4,1.0300205362462));
#17934=CARTESIAN_POINT('Origin',(0.797994444708888,0.4,1.11359995789051));
#17935=CARTESIAN_POINT('',(0.797994444708888,0.4,1.11359995789051));
#17936=CARTESIAN_POINT('',(0.797994444708888,0.4,1.11359995789051));
#17937=CARTESIAN_POINT('',(0.797994444708888,1.,1.11359995789051));
#17938=CARTESIAN_POINT('',(0.82432177520344,1.,1.09270510247943));
#17939=CARTESIAN_POINT('',(0.797994444708888,0.4,1.11359995789051));
#17940=CARTESIAN_POINT('Origin',(0.684999999999999,0.4,1.18645480318468));
#17941=CARTESIAN_POINT('',(0.684999999999999,0.4,1.18645480318468));
#17942=CARTESIAN_POINT('',(0.684999999999999,0.4,1.18645480318468));
#17943=CARTESIAN_POINT('',(0.684999999999999,1.,1.18645480318468));
#17944=CARTESIAN_POINT('',(0.71324861117722,1.,1.16824109186114));
#17945=CARTESIAN_POINT('',(0.684999999999999,0.4,1.18645480318468));
#17946=CARTESIAN_POINT('Origin',(0.56540863083202,0.4,1.24788344014201));
#17947=CARTESIAN_POINT('',(0.56540863083202,0.4,1.24788344014201));
#17948=CARTESIAN_POINT('',(0.56540863083202,0.4,1.24788344014201));
#17949=CARTESIAN_POINT('',(0.56540863083202,1.,1.24788344014201));
#17950=CARTESIAN_POINT('',(0.595306473124016,1.,1.23252628090268));
#17951=CARTESIAN_POINT('',(0.56540863083202,0.4,1.24788344014201));
#17952=CARTESIAN_POINT('Origin',(0.44037206746533,0.4,1.29729427740829));
#17953=CARTESIAN_POINT('',(0.44037206746533,0.4,1.29729427740829));
#17954=CARTESIAN_POINT('',(0.44037206746533,0.4,1.29729427740829));
#17955=CARTESIAN_POINT('',(0.44037206746533,1.,1.29729427740829));
#17956=CARTESIAN_POINT('',(0.471631208307002,1.,1.28494156809172));
#17957=CARTESIAN_POINT('',(0.44037206746533,0.4,1.29729427740829));
#17958=CARTESIAN_POINT('Origin',(0.311094480357091,0.4,1.33421146160995));
#17959=CARTESIAN_POINT('',(0.311094480357091,0.4,1.33421146160995));
#17960=CARTESIAN_POINT('',(0.311094480357091,0.4,1.33421146160995));
#17961=CARTESIAN_POINT('',(0.311094480357091,1.,1.33421146160995));
#17962=CARTESIAN_POINT('',(0.34341387713415,1.,1.32498216555953));
#17963=CARTESIAN_POINT('',(0.311094480357091,0.4,1.33421146160995));
#17964=CARTESIAN_POINT('Origin',(0.17882088334147,0.4,1.35827946008212));
#17965=CARTESIAN_POINT('',(0.17882088334147,0.4,1.35827946008212));
#17966=CARTESIAN_POINT('',(0.17882088334147,0.4,1.35827946008212));
#17967=CARTESIAN_POINT('',(0.17882088334147,1.,1.35827946008212));
#17968=CARTESIAN_POINT('',(0.211889282595374,1.,1.35226246046408));
#17969=CARTESIAN_POINT('',(0.17882088334147,0.4,1.35827946008212));
#17970=CARTESIAN_POINT('Origin',(0.104420953776041,0.4,0.793155889099048));
#17971=CARTESIAN_POINT('',(0.104420953776041,0.4,0.793155889099048));
#17972=CARTESIAN_POINT('',(0.0522104768880204,1.,0.396577944549524));
#17973=CARTESIAN_POINT('Origin',(0.527275906502257,0.4,0.913268659668847));
#17974=CARTESIAN_POINT('Origin',(0.,1.,0.));
#17975=CARTESIAN_POINT('Origin',(0.,1.,0.));
#17976=CARTESIAN_POINT('Origin',(0.,1.,0.));
#17977=CARTESIAN_POINT('Origin',(0.,1.,0.));
#17978=CARTESIAN_POINT('Origin',(0.,1.,0.));
#17979=CARTESIAN_POINT('Origin',(0.,1.,0.));
#17980=CARTESIAN_POINT('Origin',(0.,1.,0.));
#17981=CARTESIAN_POINT('Origin',(0.,1.,0.));
#17982=CARTESIAN_POINT('Origin',(0.,1.,0.));
#17983=CARTESIAN_POINT('Origin',(0.,1.,0.));
#17984=CARTESIAN_POINT('Origin',(0.,1.,0.));
#17985=CARTESIAN_POINT('Origin',(0.,1.,0.));
#17986=CARTESIAN_POINT('Origin',(0.,1.,0.));
#17987=CARTESIAN_POINT('',(-0.685,1.,1.18645480318468));
#17988=CARTESIAN_POINT('Origin',(0.,1.,0.));
#17989=CARTESIAN_POINT('',(-1.26571495954046,1.,0.524276302340173));
#17990=CARTESIAN_POINT('Origin',(0.,1.,0.));
#17991=CARTESIAN_POINT('',(-0.739103626009029,1.,0.306146745892072));
#17992=CARTESIAN_POINT('',(-0.632857479770231,1.,0.262138151170086));
#17993=CARTESIAN_POINT('',(-0.765552268585767,1.,0.23222774180357));
#17994=CARTESIAN_POINT('',(-0.745715786653214,1.,0.287666994869946));
#17995=CARTESIAN_POINT('',(-0.784628224322584,1.,0.156072257612902));
#17996=CARTESIAN_POINT('',(-0.770321257519971,1.,0.213188870755903));
#17997=CARTESIAN_POINT('',(-0.796147781337758,1.,0.0784137122636482));
#17998=CARTESIAN_POINT('',(-0.787508113576378,1.,0.136657621275589));
#17999=CARTESIAN_POINT('',(-0.8,1.,-2.22044604925031E-16));
#18000=CARTESIAN_POINT('',(-0.797110836003318,1.,0.0588102841977362));
#18001=CARTESIAN_POINT('',(-0.796147781337758,1.,-0.0784137122636487));
#18002=CARTESIAN_POINT('',(-0.799036945334439,1.,-0.0196034280659124));
#18003=CARTESIAN_POINT('',(-0.784628224322584,1.,-0.156072257612903));
#18004=CARTESIAN_POINT('',(-0.793267892083964,1.,-0.0978283486009623));
#18005=CARTESIAN_POINT('',(-0.765552268585767,1.,-0.23222774180357));
#18006=CARTESIAN_POINT('',(-0.77985923538838,1.,-0.17511112866057));
#18007=CARTESIAN_POINT('',(-0.739103626009029,1.,-0.306146745892072));
#18008=CARTESIAN_POINT('',(-0.758940107941583,1.,-0.250707492825696));
#18009=CARTESIAN_POINT('',(-1.26571495954046,1.,-0.524276302340173));
#18010=CARTESIAN_POINT('',(-0.369551813004515,1.,-0.153073372946036));
#18011=CARTESIAN_POINT('',(0.178820883341471,1.,-1.35827946008212));
#18012=CARTESIAN_POINT('Origin',(0.,1.,0.));
#18013=CARTESIAN_POINT('',(0.104420953776041,1.,-0.793155889099048));
#18014=CARTESIAN_POINT('',(0.0894104416707354,1.,-0.67913973004106));
#18015=CARTESIAN_POINT('',(0.181661010427499,1.,-0.779101583421867));
#18016=CARTESIAN_POINT('',(0.123730967938906,1.,-0.789642312679753));
#18017=CARTESIAN_POINT('',(0.257151572242529,1.,-0.757544103596084));
#18018=CARTESIAN_POINT('',(0.200533650881256,1.,-0.773712213465421));
#18019=CARTESIAN_POINT('',(0.330165623843516,1.,-0.728691059936941));
#18020=CARTESIAN_POINT('',(0.275405085142776,1.,-0.750330842681299));
#18021=CARTESIAN_POINT('',(0.4,1.,-0.692820323027551));
#18022=CARTESIAN_POINT('',(0.347624217882637,1.,-0.719723375709593));
#18023=CARTESIAN_POINT('',(0.465982157494242,1.,-0.650277347673292));
#18024=CARTESIAN_POINT('',(0.416495539373561,1.,-0.682184579188986));
#18025=CARTESIAN_POINT('',(0.527476652080055,1.,-0.601471845983182));
#18026=CARTESIAN_POINT('',(0.481355781140695,1.,-0.638075972250765));
#18027=CARTESIAN_POINT('',(0.583891258158269,1.,-0.546873841618297));
#18028=CARTESIAN_POINT('',(0.541580303599609,1.,-0.587822344891961));
#18029=CARTESIAN_POINT('',(0.634682672232988,1.,-0.487009143206976));
#18030=CARTESIAN_POINT('',(0.596589111676949,1.,-0.531907667015467));
#18031=CARTESIAN_POINT('',(1.08689407619899,1.,-0.834003157741947));
#18032=CARTESIAN_POINT('',(0.317341336116494,1.,-0.243504571603488));
#18033=CARTESIAN_POINT('Origin',(0.,1.,0.));
#18034=CARTESIAN_POINT('Origin',(0.,1.,0.));
#18035=CARTESIAN_POINT('Origin',(0.,1.,0.));
#18036=CARTESIAN_POINT('Origin',(0.,1.,0.));
#18037=CARTESIAN_POINT('Origin',(0.,1.,0.));
#18038=CARTESIAN_POINT('Origin',(-0.765552268585767,0.4,-0.23222774180357));
#18039=CARTESIAN_POINT('',(-0.765552268585767,0.4,-0.23222774180357));
#18040=CARTESIAN_POINT('',(-0.739103626009029,0.4,-0.306146745892072));
#18041=CARTESIAN_POINT('',(-0.765552268585767,0.4,-0.23222774180357));
#18042=CARTESIAN_POINT('',(-0.739103626009029,0.4,-0.306146745892072));
#18043=CARTESIAN_POINT('',(-0.765552268585767,0.4,-0.23222774180357));
#18044=CARTESIAN_POINT('Origin',(-0.784628224322584,0.4,-0.156072257612903));
#18045=CARTESIAN_POINT('',(-0.784628224322584,0.4,-0.156072257612903));
#18046=CARTESIAN_POINT('',(-0.784628224322584,0.4,-0.156072257612903));
#18047=CARTESIAN_POINT('',(-0.784628224322584,0.4,-0.156072257612903));
#18048=CARTESIAN_POINT('Origin',(-0.796147781337758,0.4,-0.0784137122636487));
#18049=CARTESIAN_POINT('',(-0.796147781337758,0.4,-0.0784137122636487));
#18050=CARTESIAN_POINT('',(-0.796147781337758,0.4,-0.0784137122636487));
#18051=CARTESIAN_POINT('',(-0.796147781337758,0.4,-0.0784137122636487));
#18052=CARTESIAN_POINT('Origin',(-0.8,0.4,-2.22044604925031E-16));
#18053=CARTESIAN_POINT('',(-0.8,0.4,-2.22044604925031E-16));
#18054=CARTESIAN_POINT('',(-0.8,0.4,-2.22044604925031E-16));
#18055=CARTESIAN_POINT('',(-0.8,0.4,-2.22044604925031E-16));
#18056=CARTESIAN_POINT('Origin',(-0.796147781337758,0.4,0.0784137122636482));
#18057=CARTESIAN_POINT('',(-0.796147781337758,0.4,0.0784137122636482));
#18058=CARTESIAN_POINT('',(-0.796147781337758,0.4,0.0784137122636482));
#18059=CARTESIAN_POINT('',(-0.796147781337758,0.4,0.0784137122636482));
#18060=CARTESIAN_POINT('Origin',(-0.784628224322584,0.4,0.156072257612902));
#18061=CARTESIAN_POINT('',(-0.784628224322584,0.4,0.156072257612902));
#18062=CARTESIAN_POINT('',(-0.784628224322584,0.4,0.156072257612902));
#18063=CARTESIAN_POINT('',(-0.784628224322584,0.4,0.156072257612902));
#18064=CARTESIAN_POINT('Origin',(-0.765552268585767,0.4,0.23222774180357));
#18065=CARTESIAN_POINT('',(-0.765552268585767,0.4,0.23222774180357));
#18066=CARTESIAN_POINT('',(-0.765552268585767,0.4,0.23222774180357));
#18067=CARTESIAN_POINT('',(-0.765552268585767,0.4,0.23222774180357));
#18068=CARTESIAN_POINT('Origin',(-0.739103626009029,0.4,0.306146745892072));
#18069=CARTESIAN_POINT('',(-0.739103626009029,0.4,0.306146745892072));
#18070=CARTESIAN_POINT('',(-0.739103626009029,0.4,0.306146745892072));
#18071=CARTESIAN_POINT('',(-0.739103626009029,0.4,0.306146745892072));
#18072=CARTESIAN_POINT('Origin',(-1.26571495954046,0.4,0.524276302340173));
#18073=CARTESIAN_POINT('',(-1.26571495954046,0.4,0.524276302340173));
#18074=CARTESIAN_POINT('',(-1.26571495954046,0.4,0.524276302340173));
#18075=CARTESIAN_POINT('',(-1.26571495954046,0.4,0.524276302340173));
#18076=CARTESIAN_POINT('Origin',(-1.31100825995313,0.4,0.397690007838613));
#18077=CARTESIAN_POINT('',(-1.31100825995313,0.4,0.397690007838613));
#18078=CARTESIAN_POINT('',(-1.31100825995313,0.4,0.397690007838613));
#18079=CARTESIAN_POINT('',(-1.31100825995313,1.,0.397690007838613));
#18080=CARTESIAN_POINT('',(-1.29968493484996,1.,0.429336581464004));
#18081=CARTESIAN_POINT('',(-1.31100825995313,0.4,0.397690007838613));
#18082=CARTESIAN_POINT('Origin',(-1.34367583415243,0.4,0.267273741162095));
#18083=CARTESIAN_POINT('',(-1.34367583415243,0.4,0.267273741162095));
#18084=CARTESIAN_POINT('',(-1.34367583415243,0.4,0.267273741162095));
#18085=CARTESIAN_POINT('',(-1.34367583415243,1.,0.267273741162095));
#18086=CARTESIAN_POINT('',(-1.3355089406026,1.,0.299877807831225));
#18087=CARTESIAN_POINT('',(-1.34367583415243,0.4,0.267273741162095));
#18088=CARTESIAN_POINT('Origin',(-1.36340307554091,0.4,0.134283482251498));
#18089=CARTESIAN_POINT('',(-1.36340307554091,0.4,0.134283482251498));
#18090=CARTESIAN_POINT('',(-1.36340307554091,0.4,0.134283482251498));
#18091=CARTESIAN_POINT('',(-1.36340307554091,1.,0.134283482251498));
#18092=CARTESIAN_POINT('',(-1.35847126519379,1.,0.167531046979148));
#18093=CARTESIAN_POINT('',(-1.36340307554091,0.4,0.134283482251498));
#18094=CARTESIAN_POINT('Origin',(-1.37,0.4,-3.33066907387547E-16));
#18095=CARTESIAN_POINT('',(-1.37,0.4,-3.33066907387547E-16));
#18096=CARTESIAN_POINT('',(-1.37,0.4,-3.33066907387547E-16));
#18097=CARTESIAN_POINT('',(-1.37,1.,-3.33066907387547E-16));
#18098=CARTESIAN_POINT('',(-1.36835076888523,1.,0.0335708705628729));
#18099=CARTESIAN_POINT('',(-1.37,0.4,-3.33066907387547E-16));
#18100=CARTESIAN_POINT('Origin',(-1.36340307554091,0.4,-0.134283482251498));
#18101=CARTESIAN_POINT('',(-1.36340307554091,0.4,-0.134283482251498));
#18102=CARTESIAN_POINT('',(-1.36340307554091,0.4,-0.134283482251498));
#18103=CARTESIAN_POINT('',(-1.36340307554091,1.,-0.134283482251498));
#18104=CARTESIAN_POINT('',(-1.36505230665568,1.,-0.100712611688622));
#18105=CARTESIAN_POINT('',(-1.36340307554091,0.4,-0.134283482251498));
#18106=CARTESIAN_POINT('Origin',(-1.34367583415243,0.4,-0.267273741162096));
#18107=CARTESIAN_POINT('',(-1.34367583415243,0.4,-0.267273741162096));
#18108=CARTESIAN_POINT('',(-1.34367583415243,0.4,-0.267273741162096));
#18109=CARTESIAN_POINT('',(-1.34367583415243,1.,-0.267273741162096));
#18110=CARTESIAN_POINT('',(-1.34860764449955,1.,-0.234026176434447));
#18111=CARTESIAN_POINT('',(-1.34367583415243,0.4,-0.267273741162096));
#18112=CARTESIAN_POINT('Origin',(-1.31100825995313,0.4,-0.397690007838614));
#18113=CARTESIAN_POINT('',(-1.31100825995313,0.4,-0.397690007838614));
#18114=CARTESIAN_POINT('',(-1.31100825995313,0.4,-0.397690007838614));
#18115=CARTESIAN_POINT('',(-1.31100825995313,1.,-0.397690007838614));
#18116=CARTESIAN_POINT('',(-1.31917515350295,1.,-0.365085941169485));
#18117=CARTESIAN_POINT('',(-1.31100825995313,0.4,-0.397690007838614));
#18118=CARTESIAN_POINT('Origin',(-1.26571495954046,0.4,-0.524276302340173));
#18119=CARTESIAN_POINT('',(-1.26571495954046,0.4,-0.524276302340173));
#18120=CARTESIAN_POINT('',(-1.26571495954046,0.4,-0.524276302340173));
#18121=CARTESIAN_POINT('',(-1.27703828464363,1.,-0.492629728714784));
#18122=CARTESIAN_POINT('',(-1.26571495954046,0.4,-0.524276302340173));
#18123=CARTESIAN_POINT('Origin',(-0.739103626009029,0.4,-0.306146745892072));
#18124=CARTESIAN_POINT('',(-0.739103626009029,0.4,-0.306146745892072));
#18125=CARTESIAN_POINT('Origin',(-1.05455181300451,0.4,-3.33066907387547E-16));
#18126=CARTESIAN_POINT('Origin',(0.,1.,0.));
#18127=CARTESIAN_POINT('Origin',(0.,1.,0.));
#18128=CARTESIAN_POINT('Origin',(0.,1.,0.));
#18129=CARTESIAN_POINT('Origin',(0.,1.,0.));
#18130=CARTESIAN_POINT('Origin',(0.,1.,0.));
#18131=CARTESIAN_POINT('Origin',(0.,1.,0.));
#18132=CARTESIAN_POINT('Origin',(0.,1.,0.));
#18133=CARTESIAN_POINT('Origin',(0.,1.,0.));
#18134=CARTESIAN_POINT('Origin',(0.,1.,0.));
#18135=CARTESIAN_POINT('Origin',(0.,1.,0.));
#18136=CARTESIAN_POINT('Origin',(0.,1.,0.));
#18137=CARTESIAN_POINT('Origin',(0.,1.,0.));
#18138=CARTESIAN_POINT('Origin',(0.,1.,0.));
#18139=CARTESIAN_POINT('Origin',(0.,1.,0.));
#18140=CARTESIAN_POINT('Origin',(0.,1.,0.));
#18141=CARTESIAN_POINT('Origin',(0.,1.,0.));
#18142=CARTESIAN_POINT('Origin',(0.583891258158269,0.4,-0.546873841618297));
#18143=CARTESIAN_POINT('',(0.583891258158269,0.4,-0.546873841618297));
#18144=CARTESIAN_POINT('',(0.634682672232988,0.4,-0.487009143206976));
#18145=CARTESIAN_POINT('',(0.583891258158269,0.4,-0.546873841618297));
#18146=CARTESIAN_POINT('',(0.634682672232988,0.4,-0.487009143206976));
#18147=CARTESIAN_POINT('',(0.583891258158269,0.4,-0.546873841618297));
#18148=CARTESIAN_POINT('Origin',(0.527476652080055,0.4,-0.601471845983182));
#18149=CARTESIAN_POINT('',(0.527476652080055,0.4,-0.601471845983182));
#18150=CARTESIAN_POINT('',(0.527476652080055,0.4,-0.601471845983182));
#18151=CARTESIAN_POINT('',(0.527476652080055,0.4,-0.601471845983182));
#18152=CARTESIAN_POINT('Origin',(0.465982157494242,0.4,-0.650277347673292));
#18153=CARTESIAN_POINT('',(0.465982157494242,0.4,-0.650277347673292));
#18154=CARTESIAN_POINT('',(0.465982157494242,0.4,-0.650277347673292));
#18155=CARTESIAN_POINT('',(0.465982157494242,0.4,-0.650277347673292));
#18156=CARTESIAN_POINT('Origin',(0.4,0.4,-0.692820323027551));
#18157=CARTESIAN_POINT('',(0.4,0.4,-0.692820323027551));
#18158=CARTESIAN_POINT('',(0.4,0.4,-0.692820323027551));
#18159=CARTESIAN_POINT('',(0.4,0.4,-0.692820323027551));
#18160=CARTESIAN_POINT('Origin',(0.330165623843516,0.4,-0.728691059936941));
#18161=CARTESIAN_POINT('',(0.330165623843516,0.4,-0.728691059936941));
#18162=CARTESIAN_POINT('',(0.330165623843516,0.4,-0.728691059936941));
#18163=CARTESIAN_POINT('',(0.330165623843516,0.4,-0.728691059936941));
#18164=CARTESIAN_POINT('Origin',(0.257151572242529,0.4,-0.757544103596084));
#18165=CARTESIAN_POINT('',(0.257151572242529,0.4,-0.757544103596084));
#18166=CARTESIAN_POINT('',(0.257151572242529,0.4,-0.757544103596084));
#18167=CARTESIAN_POINT('',(0.257151572242529,0.4,-0.757544103596084));
#18168=CARTESIAN_POINT('Origin',(0.181661010427499,0.4,-0.779101583421867));
#18169=CARTESIAN_POINT('',(0.181661010427499,0.4,-0.779101583421867));
#18170=CARTESIAN_POINT('',(0.181661010427499,0.4,-0.779101583421867));
#18171=CARTESIAN_POINT('',(0.181661010427499,0.4,-0.779101583421867));
#18172=CARTESIAN_POINT('Origin',(0.104420953776041,0.4,-0.793155889099048));
#18173=CARTESIAN_POINT('',(0.104420953776041,0.4,-0.793155889099048));
#18174=CARTESIAN_POINT('',(0.104420953776041,0.4,-0.793155889099048));
#18175=CARTESIAN_POINT('',(0.104420953776041,0.4,-0.793155889099048));
#18176=CARTESIAN_POINT('Origin',(0.178820883341471,0.4,-1.35827946008212));
#18177=CARTESIAN_POINT('',(0.178820883341471,0.4,-1.35827946008212));
#18178=CARTESIAN_POINT('',(0.178820883341471,0.4,-1.35827946008212));
#18179=CARTESIAN_POINT('',(0.178820883341471,0.4,-1.35827946008212));
#18180=CARTESIAN_POINT('Origin',(0.311094480357091,0.4,-1.33421146160995));
#18181=CARTESIAN_POINT('',(0.311094480357091,0.4,-1.33421146160995));
#18182=CARTESIAN_POINT('',(0.311094480357091,0.4,-1.33421146160995));
#18183=CARTESIAN_POINT('',(0.311094480357092,1.,-1.33421146160995));
#18184=CARTESIAN_POINT('',(0.278026081103186,1.,-1.34022846122799));
#18185=CARTESIAN_POINT('',(0.311094480357091,0.4,-1.33421146160995));
#18186=CARTESIAN_POINT('Origin',(0.440372067465332,0.4,-1.29729427740829));
#18187=CARTESIAN_POINT('',(0.440372067465332,0.4,-1.29729427740829));
#18188=CARTESIAN_POINT('',(0.440372067465332,0.4,-1.29729427740829));
#18189=CARTESIAN_POINT('',(0.440372067465332,1.,-1.29729427740829));
#18190=CARTESIAN_POINT('',(0.408052670688271,1.,-1.30652357345871));
#18191=CARTESIAN_POINT('',(0.440372067465332,0.4,-1.29729427740829));
#18192=CARTESIAN_POINT('Origin',(0.565408630832021,0.4,-1.24788344014201));
#18193=CARTESIAN_POINT('',(0.565408630832021,0.4,-1.24788344014201));
#18194=CARTESIAN_POINT('',(0.565408630832021,0.4,-1.24788344014201));
#18195=CARTESIAN_POINT('',(0.565408630832021,1.,-1.24788344014201));
#18196=CARTESIAN_POINT('',(0.534149489990348,1.,-1.26023614945858));
#18197=CARTESIAN_POINT('',(0.565408630832021,0.4,-1.24788344014201));
#18198=CARTESIAN_POINT('Origin',(0.685,0.4,-1.18645480318468));
#18199=CARTESIAN_POINT('',(0.685,0.4,-1.18645480318468));
#18200=CARTESIAN_POINT('',(0.685,0.4,-1.18645480318468));
#18201=CARTESIAN_POINT('',(0.685,1.,-1.18645480318468));
#18202=CARTESIAN_POINT('',(0.655102157708007,1.,-1.20181196242401));
#18203=CARTESIAN_POINT('',(0.685,0.4,-1.18645480318468));
#18204=CARTESIAN_POINT('Origin',(0.797994444708889,0.4,-1.11359995789051));
#18205=CARTESIAN_POINT('',(0.797994444708889,0.4,-1.11359995789051));
#18206=CARTESIAN_POINT('',(0.797994444708889,0.4,-1.11359995789051));
#18207=CARTESIAN_POINT('',(0.797994444708889,1.,-1.11359995789051));
#18208=CARTESIAN_POINT('',(0.769745833531666,1.,-1.13181366921406));
#18209=CARTESIAN_POINT('',(0.797994444708889,0.4,-1.11359995789051));
#18210=CARTESIAN_POINT('Origin',(0.903303766687094,0.4,-1.0300205362462));
#18211=CARTESIAN_POINT('',(0.903303766687094,0.4,-1.0300205362462));
#18212=CARTESIAN_POINT('',(0.903303766687094,0.4,-1.0300205362462));
#18213=CARTESIAN_POINT('',(0.903303766687094,1.,-1.0300205362462));
#18214=CARTESIAN_POINT('',(0.876976436192544,1.,-1.05091539165728));
#18215=CARTESIAN_POINT('',(0.903303766687094,0.4,-1.0300205362462));
#18216=CARTESIAN_POINT('Origin',(0.999913779596035,0.4,-0.936521453771333));
#18217=CARTESIAN_POINT('',(0.999913779596035,0.4,-0.936521453771333));
#18218=CARTESIAN_POINT('',(0.999913779596035,0.4,-0.936521453771333));
#18219=CARTESIAN_POINT('',(0.999913779596035,1.,-0.936521453771333));
#18220=CARTESIAN_POINT('',(0.9757612763688,1.,-0.959896224390049));
#18221=CARTESIAN_POINT('',(0.999913779596035,0.4,-0.936521453771333));
#18222=CARTESIAN_POINT('Origin',(1.08689407619899,0.4,-0.834003157741947));
#18223=CARTESIAN_POINT('',(1.08689407619899,0.4,-0.834003157741947));
#18224=CARTESIAN_POINT('',(1.08689407619899,0.4,-0.834003157741947));
#18225=CARTESIAN_POINT('',(1.06514900204825,1.,-0.859632731749293));
#18226=CARTESIAN_POINT('',(1.08689407619899,0.4,-0.834003157741947));
#18227=CARTESIAN_POINT('Origin',(0.634682672232988,0.4,-0.487009143206976));
#18228=CARTESIAN_POINT('',(0.634682672232988,0.4,-0.487009143206976));
#18229=CARTESIAN_POINT('Origin',(0.527275906502257,0.4,-0.913268659668847));
#18230=CARTESIAN_POINT('Origin',(0.,1.,0.));
#18231=CARTESIAN_POINT('Origin',(0.,1.,0.));
#18232=CARTESIAN_POINT('Origin',(0.,1.,0.));
#18233=CARTESIAN_POINT('Origin',(0.,1.,0.));
#18234=CARTESIAN_POINT('Origin',(0.,1.,0.));
#18235=CARTESIAN_POINT('Origin',(0.,1.,0.));
#18236=CARTESIAN_POINT('Origin',(0.,1.,0.));
#18237=CARTESIAN_POINT('Origin',(0.,1.,0.));
#18238=CARTESIAN_POINT('Origin',(0.,1.,0.));
#18239=CARTESIAN_POINT('Origin',(0.,1.,0.));
#18240=CARTESIAN_POINT('Origin',(0.,1.,0.));
#18241=CARTESIAN_POINT('Origin',(0.,1.,0.));
#18242=CARTESIAN_POINT('Origin',(0.,1.,0.));
#18243=CARTESIAN_POINT('Origin',(0.,1.,0.));
#18244=CARTESIAN_POINT('Origin',(0.,1.,0.));
#18245=CARTESIAN_POINT('Origin',(0.,1.,0.));
#18246=CARTESIAN_POINT('Origin',(0.,1.,0.));
#18247=CARTESIAN_POINT('',(-0.685,2.05,1.18645480318468));
#18248=CARTESIAN_POINT('Origin',(0.,2.05,0.));
#18249=CARTESIAN_POINT('',(-0.685,1.,1.18645480318468));
#18250=CARTESIAN_POINT('Origin',(0.,2.05,0.));
#19318=UNCERTAINTY_MEASURE_WITH_UNIT(LENGTH_MEASURE(0.001),#19362,
'DISTANCE_ACCURACY_VALUE',
'Maximum model space distance between geometric entities at asserted c
onnectivities');
#19323=UNCERTAINTY_MEASURE_WITH_UNIT(LENGTH_MEASURE(0.001),#19362,
'DISTANCE_ACCURACY_VALUE',
'Maximum model space distance between geometric entities at asserted c
onnectivities');
#19356=(
GEOMETRIC_REPRESENTATION_CONTEXT(3)
GLOBAL_UNCERTAINTY_ASSIGNED_CONTEXT((#19318))
GLOBAL_UNIT_ASSIGNED_CONTEXT((#19362,#19364,#19365))
REPRESENTATION_CONTEXT('','3D')
);
#19361=(
GEOMETRIC_REPRESENTATION_CONTEXT(3)
GLOBAL_UNCERTAINTY_ASSIGNED_CONTEXT((#19323))
GLOBAL_UNIT_ASSIGNED_CONTEXT((#19362,#19364,#19365))
REPRESENTATION_CONTEXT('','3D')
);
#19362=(
LENGTH_UNIT()
NAMED_UNIT(*)
SI_UNIT(.CENTI.,.METRE.)
);
#19364=(
NAMED_UNIT(*)
PLANE_ANGLE_UNIT()
SI_UNIT($,.RADIAN.)
);
#19365=(
NAMED_UNIT(*)
SI_UNIT($,.STERADIAN.)
SOLID_ANGLE_UNIT()
);
#19398=SHAPE_DEFINITION_REPRESENTATION(#19462,#19520);
#19462=PRODUCT_DEFINITION_SHAPE('',$,#19558);
#19520=SHAPE_REPRESENTATION('',(#11982),#19356);
#19525=PRODUCT_DEFINITION_CONTEXT('part definition',#19638,'design');
#19558=PRODUCT_DEFINITION('Hub B','Hub B',#19595,#19525);
#19595=PRODUCT_DEFINITION_FORMATION('',$,#19672);
#19638=APPLICATION_CONTEXT(
'Core Data for Automotive Mechanical Design Process');
#19639=PRODUCT_CONTEXT('part definition',#19638,'mechanical');
#19672=PRODUCT('Hub B','Hub B','Hub B',(#19639));
#19733=COLOUR_RGB('Sky Blue',0.24,0.69,0.87);
#19734=FILL_AREA_STYLE_COLOUR('',#19733);
#19735=FILL_AREA_STYLE('',(#19734));
#19736=SURFACE_STYLE_FILL_AREA(#19735);
#19737=SURFACE_SIDE_STYLE('',(#19736));
#19738=SURFACE_STYLE_USAGE(.BOTH.,#19737);
#19739=PRESENTATION_STYLE_ASSIGNMENT((#19738));
ENDSEC;
END-ISO-10303-21;
